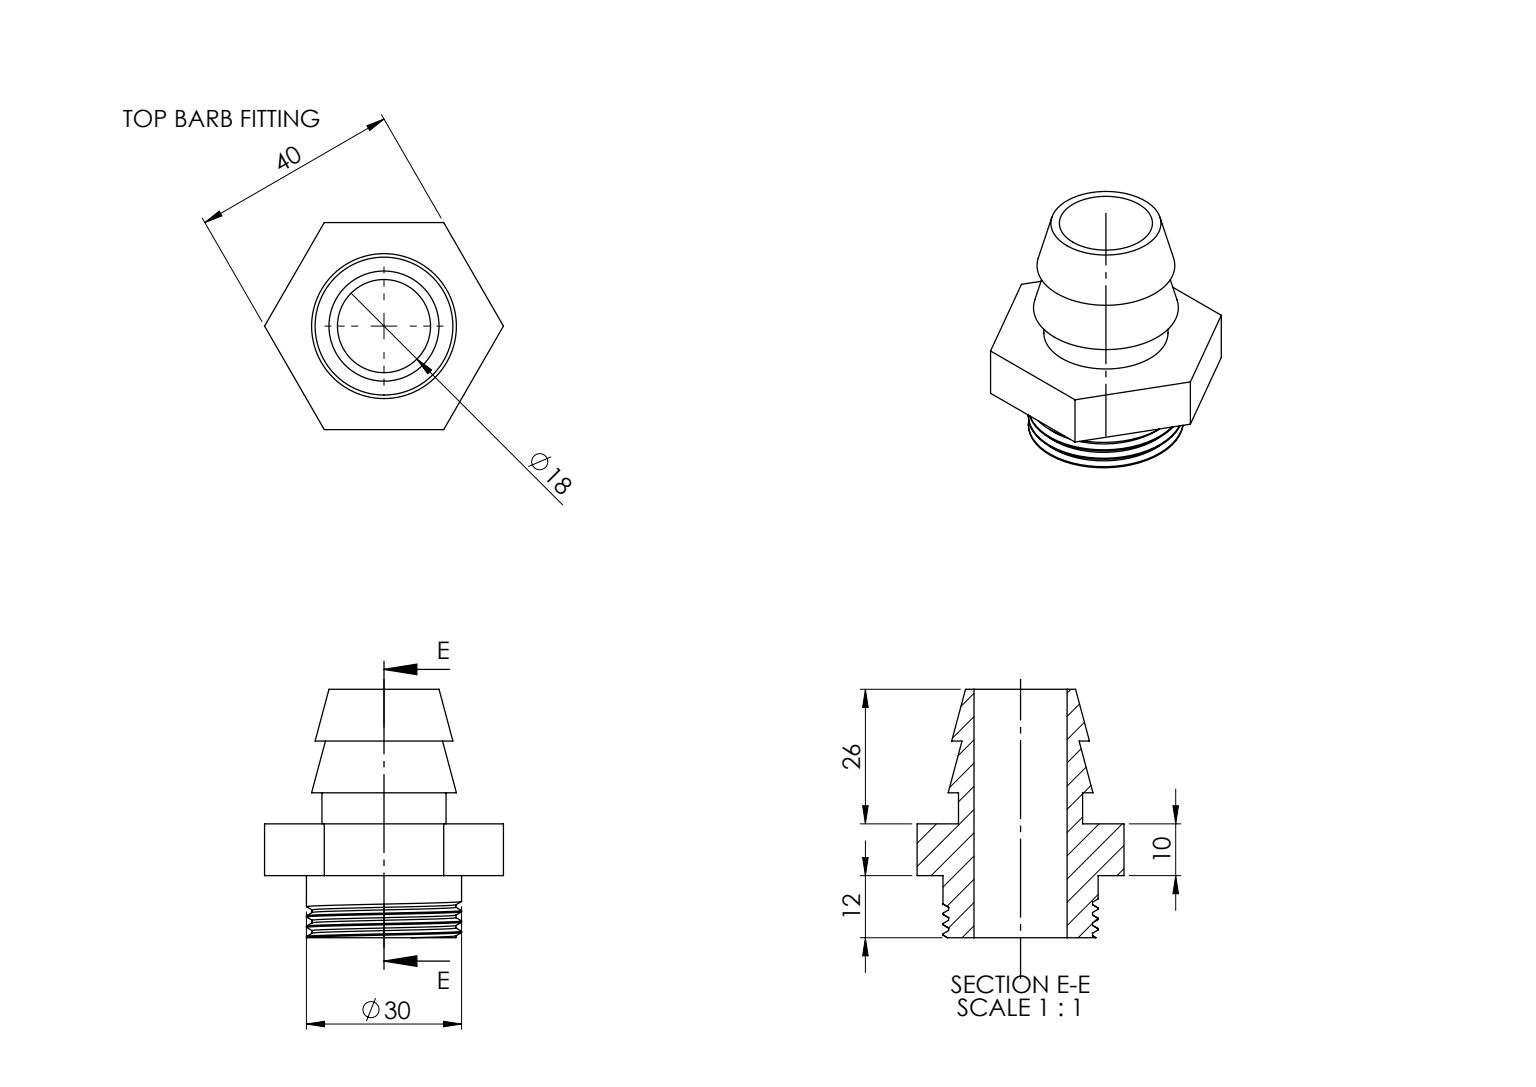
ISO-10303-21;
HEADER;
FILE_DESCRIPTION (('STEP AP214'),
    '1' );
FILE_NAME ('top barb fitting.step',
    '2026-10-02T18:08:48',
    ( '' ),
    ( '' ),
    'SwSTEP 2.0',
    'SolidWorks 2026',
    '' );
FILE_SCHEMA (( 'AUTOMOTIVE_DESIGN' ));
ENDSEC;

DATA;
#6=B_SPLINE_CURVE_WITH_KNOTS ( 'NONE', 3,
 ( #2746, #31563, #23520, #5150, #31895, #33979, #26595, #13563, #7891, #10812, #8061, #21292, #8391, #3092, #18876, #13210, #18378, #13388, #5322, #18546, #24026, #325, #29325, #15802, #5827, #26258, #31732, #495, #23687, #16306, #152, #15636, #2584, #10642 ),
 .UNSPECIFIED., .F., .F.,
 ( 4, 2, 2, 2, 2, 2, 2, 2, 2, 2, 2, 2, 2, 2, 2, 2, 4 ),
 ( 6.762863467562367515E-16, 0.001783076374787156146, 0.003566152749573635750, 0.007132305499146594091, 0.008023843686539834652, 0.008915381873933073478, 0.01069845824871955460, 0.01248153462350603572, 0.01426461099829251858, 0.01604768737307899970, 0.01783076374786548429, 0.02139691649743844307, 0.02228845468483168710, 0.02317999287222492766, 0.02496306924701141225, 0.02674614562179789337, 0.02852922199658437796 ),
 .UNSPECIFIED. ) ;
#9=CARTESIAN_POINT ( 'NONE',  ( -23.09401076758502924, 96.00000000000002842, 5.354274672883389237E-15 ) ) ;
#12=PRODUCT ( 'top barb fitting', 'top barb fitting', '', ( #25356 ) ) ;
#18=CARTESIAN_POINT ( 'NONE',  ( 13.91687918246660871, 74.00000000000008527, 0.9182373085827880699 ) ) ;
#119=DIRECTION ( 'NONE',  ( -0.000000000000000000, 1.000000000000000000, -0.000000000000000000 ) ) ;
#130=EDGE_LOOP ( 'NONE', ( #13807, #32440, #5639, #27881 ) ) ;
#142=CARTESIAN_POINT ( 'NONE',  ( -15.00000000000000000, 72.09999999999999432, 4.873795443493597723 ) ) ;
#152=CARTESIAN_POINT ( 'NONE',  ( 11.86847005202517380, 74.00000000000004263, -7.471229617278120294 ) ) ;
#163=CARTESIAN_POINT ( 'NONE',  ( 8.601468415847520532, 79.57500000273117280, 11.83890561707634603 ) ) ;
#166=CARTESIAN_POINT ( 'NONE',  ( 8.601468415847516980, 76.67500000273118133, -11.83890561707634781 ) ) ;
#187=AXIS2_PLACEMENT_3D ( 'NONE', #2552, #20584, #13357 ) ;
#196=CARTESIAN_POINT ( 'NONE',  ( -1.714505518806294835E-15, 102.0000000000000284, -14.00000000000000178 ) ) ;
#220=VERTEX_POINT ( 'NONE', #33464 ) ;
#287=CARTESIAN_POINT ( 'NONE',  ( 15.00000000000000355, 71.15000000546237402, 4.873795443493592394 ) ) ;
#293=ADVANCED_FACE ( 'NONE', ( #15638 ), #7725, .F. ) ;
#325=CARTESIAN_POINT ( 'NONE',  ( 6.987025175984479475, 74.00000000000002842, -12.51940829596972016 ) ) ;
#333=DIRECTION ( 'NONE',  ( -0.000000000000000000, -1.000000000000000000, -0.000000000000000000 ) ) ;
#335=CARTESIAN_POINT ( 'NONE',  ( 0.000000000000000000, 74.00000000000001421, 0.000000000000000000 ) ) ;
#338=CARTESIAN_POINT ( 'NONE',  ( -4.300734207923759378, 76.47500000273116427, -13.23629886949340495 ) ) ;
#341=CARTESIAN_POINT ( 'NONE',  ( -13.91746824999999887, 75.37500000273116996, 0.000000000000000000 ) ) ;
#357=CARTESIAN_POINT ( 'NONE',  ( -11.25946833292375793, 77.17500000273119554, -8.180482586598733619 ) ) ;
#432=CARTESIAN_POINT ( 'NONE',  ( 1.836970198721029589E-15, 86.00000000000001421, -15.00000000000000000 ) ) ;
#459=CARTESIAN_POINT ( 'NONE',  ( 2.688165632520823219E-15, 79.37500000273116996, 14.63369212191046387 ) ) ;
#486=CARTESIAN_POINT ( 'NONE',  ( -15.00000000000000000, 72.00000000000001421, 0.000000000000000000 ) ) ;
#495=CARTESIAN_POINT ( 'NONE',  ( 10.52536686629071916, 74.00000000000000000, -9.403734997071314439 ) ) ;
#507=CARTESIAN_POINT ( 'NONE',  ( 4.300734207923761154, 77.47500000273116427, 13.23629886949340495 ) ) ;
#510=CARTESIAN_POINT ( 'NONE',  ( 11.25946833292375793, 72.17500000273119554, 8.180482586598731842 ) ) ;
#523=CARTESIAN_POINT ( 'NONE',  ( 11.25946833292375793, 78.17500000273119554, 8.180482586598731842 ) ) ;
#527=CARTESIAN_POINT ( 'NONE',  ( 13.03261263866114206, 74.00000000000001421, 4.904499419084999090 ) ) ;
#550=CARTESIAN_POINT ( 'NONE',  ( -11.25946833292375793, 80.67500000273119554, -8.180482586598733619 ) ) ;
#612=CARTESIAN_POINT ( 'NONE',  ( -1.089172066684569321E-14, 76.75000000546238255, 15.00000000000000000 ) ) ;
#623=CARTESIAN_POINT ( 'NONE',  ( -8.601468415847518756, 78.57500000273120122, -11.83890561707634781 ) ) ;
#647=CARTESIAN_POINT ( 'NONE',  ( 1.836970198721029589E-15, 74.00000000000001421, -15.00000000000000000 ) ) ;
#651=CARTESIAN_POINT ( 'NONE',  ( -12.13525491562420910, 72.19999999999998863, 8.816778784387098611 ) ) ;
#691=CARTESIAN_POINT ( 'NONE',  ( -11.25946833292375793, 79.57500000273121543, 8.180482586598737171 ) ) ;
#716=CARTESIAN_POINT ( 'NONE',  ( -13.91746824999999887, 78.87500000273118417, 0.000000000000000000 ) ) ;
#728=AXIS2_PLACEMENT_3D ( 'NONE', #8070, #26267, #31742 ) ;
#731=LINE ( 'NONE', #16213, #1228 ) ;
#743=ORIENTED_EDGE ( 'NONE', *, *, #12358, .F. ) ;
#754=AXIS2_PLACEMENT_3D ( 'NONE', #32475, #1069, #27509 ) ;
#759=DIRECTION ( 'NONE',  ( -0.000000000000000000, 1.000000000000000000, -0.000000000000000000 ) ) ;
#777=CARTESIAN_POINT ( 'NONE',  ( 15.00000000000000000, 75.35000000546236265, -4.873795443493596835 ) ) ;
#784=CARTESIAN_POINT ( 'NONE',  ( -8.891200544363830713E-16, 77.75000000546235412, -15.00000000000000000 ) ) ;
#792=CARTESIAN_POINT ( 'NONE',  ( 8.601468415847516980, 80.17500000273113869, -11.83890561707634781 ) ) ;
#797=CARTESIAN_POINT ( 'NONE',  ( -15.00000000000000000, 80.15000000546237402, -4.873795443493594171 ) ) ;
#818=COLOUR_RGB ( '', 0.40784314, 0.44705882, 0.49803922) ;
#852=AXIS2_PLACEMENT_3D ( 'NONE', #3223, #24155, #11436 ) ;
#858=CARTESIAN_POINT ( 'NONE',  ( -8.601468415847518756, 81.07500000273115859, -11.83890561707634781 ) ) ;
#865=DIRECTION ( 'NONE',  ( -0.5000000000000002220, 0.000000000000000000, -0.8660254037844384856 ) ) ;
#866=CARTESIAN_POINT ( 'NONE',  ( -11.25946833292375793, 75.57500000273120122, 8.180482586598737171 ) ) ;
#868=FACE_OUTER_BOUND ( 'NONE', #18191, .T. ) ;
#871=VERTEX_POINT ( 'NONE', #20231 ) ;
#874=CARTESIAN_POINT ( 'NONE',  ( -14.45873412499999944, 81.68750000136559208, 0.000000000000000000 ) ) ;
#883=CARTESIAN_POINT ( 'NONE',  ( -11.25946833292375793, 79.07500000273121543, 8.180482586598737171 ) ) ;
#893=EDGE_LOOP ( 'NONE', ( #32042, #24575 ) ) ;
#921=CARTESIAN_POINT ( 'NONE',  ( 0.000000000000000000, 111.9999999999999858, 0.000000000000000000 ) ) ;
#953=CARTESIAN_POINT ( 'NONE',  ( 11.25946833292375793, 75.67500000273119554, 8.180482586598731842 ) ) ;
#1003=CARTESIAN_POINT ( 'NONE',  ( -4.300734207923755825, 71.77500000273117564, 13.23629886949340673 ) ) ;
#1004=DIRECTION ( 'NONE',  ( -0.000000000000000000, -1.000000000000000000, -0.000000000000000000 ) ) ;
#1016=CARTESIAN_POINT ( 'NONE',  ( -12.13525491562421088, 81.79999999999998295, -8.816778784387096835 ) ) ;
#1027=CARTESIAN_POINT ( 'NONE',  ( -13.91746824999999887, 79.37500000273118417, 0.000000000000000000 ) ) ;
#1043=CARTESIAN_POINT ( 'NONE',  ( 8.601468415847520532, 77.57500000273115859, 11.83890561707634781 ) ) ;
#1069=DIRECTION ( 'NONE',  ( 0.000000000000000000, 1.000000000000000000, 0.000000000000000000 ) ) ;
#1099=CARTESIAN_POINT ( 'NONE',  ( 2.375766604868046361, 74.80125428700921475, 14.99999999999999822 ) ) ;
#1105=CARTESIAN_POINT ( 'NONE',  ( -8.891200544363830713E-16, 77.49999999999998579, -15.00000000000000000 ) ) ;
#1113=CARTESIAN_POINT ( 'NONE',  ( -13.91746824999999532, 76.97500000273119269, 4.522059556121122093 ) ) ;
#1186=CARTESIAN_POINT ( 'NONE',  ( 13.91746825000000065, 72.27500000273116143, 4.522059556121114987 ) ) ;
#1196=CARTESIAN_POINT ( 'NONE',  ( -11.25946833292375793, 77.17500000273119554, -8.180482586598733619 ) ) ;
#1210=CARTESIAN_POINT ( 'NONE',  ( -4.300734207923755825, 79.27500000273118985, 13.23629886949340673 ) ) ;
#1228=VECTOR ( 'NONE', #21690, 1000.000000000000114 ) ;
#1250=CARTESIAN_POINT ( 'NONE',  ( -13.91746824999999532, 80.77500000273118985, -4.522059556121115875 ) ) ;
#1253=FILL_AREA_STYLE ('',( #27360 ) ) ;
#1256=ADVANCED_FACE ( 'NONE', ( #33351, #25805 ), #9849, .F. ) ;
#1262=ADVANCED_FACE ( 'NONE', ( #28543, #2297 ), #10028, .T. ) ;
#1269=CARTESIAN_POINT ( 'NONE',  ( -4.635254915624211769, 75.59999999999999432, -14.26584774442730286 ) ) ;
#1285=CARTESIAN_POINT ( 'NONE',  ( -8.601468415847518756, 74.57500000273120122, -11.83890561707634781 ) ) ;
#1300=CLOSED_SHELL ( 'NONE', ( #7560, #13574, #15897, #13035, #6079, #19634, #15027, #28982, #8831, #17642, #33557, #1262, #15751, #14298, #30209, #23775, #26972, #23633, #2088, #3006, #29689, #33907, #4803, #9146, #33895, #7895, #1256, #14876, #293, #28324, #14823, #26573 ) ) ;
#1315=CARTESIAN_POINT ( 'NONE',  ( -3.922490400387641962, 74.00000000000000000, 13.75156615976576902 ) ) ;
#1320=( NAMED_UNIT ( * ) SI_UNIT ( $, .STERADIAN. ) SOLID_ANGLE_UNIT ( ) );
#1338=CARTESIAN_POINT ( 'NONE',  ( -12.13525491562420910, 78.45000000546237118, 8.816778784387098611 ) ) ;
#1348=VECTOR ( 'NONE', #1004, 1000.000000000000000 ) ;
#1358=CARTESIAN_POINT ( 'NONE',  ( -8.960552108402742093E-16, 74.87500000273119838, -14.63369212191046387 ) ) ;
#1368=AXIS2_PLACEMENT_3D ( 'NONE', #32981, #17395, #27514 ) ;
#1370=CARTESIAN_POINT ( 'NONE',  ( -4.300734207923759378, 80.97500000273122112, -13.23629886949340495 ) ) ;
#1372=CARTESIAN_POINT ( 'NONE',  ( -4.635254915624211769, 77.85000000546237686, -14.26584774442730286 ) ) ;
#1376=AXIS2_PLACEMENT_3D ( 'NONE', #6186, #27460, #21818 ) ;
#1387=CARTESIAN_POINT ( 'NONE',  ( 8.601468415847520532, 71.57500000273118701, 11.83890561707634781 ) ) ;
#1437=AXIS2_PLACEMENT_3D ( 'NONE', #30037, #32278, #3798 ) ;
#1459=CARTESIAN_POINT ( 'NONE',  ( 13.91746824999999532, 73.97500000273115006, -4.522059556121118540 ) ) ;
#1470=VECTOR ( 'NONE', #27620, 1000.000000000000000 ) ;
#1509=CARTESIAN_POINT ( 'NONE',  ( -15.00000000000000000, 78.25000000546239676, 0.000000000000000000 ) ) ;
#1517=ORIENTED_EDGE ( 'NONE', *, *, #21552, .F. ) ;
#1530=CARTESIAN_POINT ( 'NONE',  ( 13.91746824999999532, 72.47500000273116427, -4.522059556121118540 ) ) ;
#1541=CARTESIAN_POINT ( 'NONE',  ( 4.635254915624209993, 77.65000000546234560, -14.26584774442730463 ) ) ;
#1553=CARTESIAN_POINT ( 'NONE',  ( -8.960552108402742093E-16, 80.87500000273116996, -14.63369212191046387 ) ) ;
#1624=CARTESIAN_POINT ( 'NONE',  ( 8.601468415847516980, 76.17500000273115290, -11.83890561707634781 ) ) ;
#1644=EDGE_CURVE ( 'NONE', #17496, #30053, #15696, .T. ) ;
#1699=CARTESIAN_POINT ( 'NONE',  ( 4.300734207923757602, 72.77500000273118985, -13.23629886949340673 ) ) ;
#1710=CARTESIAN_POINT ( 'NONE',  ( 12.13525491562421088, 77.05000000546242234, 8.816778784387095058 ) ) ;
#1722=CARTESIAN_POINT ( 'NONE',  ( 4.300734207923757602, 80.77500000273118985, -13.23629886949340673 ) ) ;
#1724=LINE ( 'NONE', #12204, #13775 ) ;
#1792=FACE_OUTER_BOUND ( 'NONE', #13191, .T. ) ;
#1798=CARTESIAN_POINT ( 'NONE',  ( -8.601468415847515203, 71.17500000273118133, 11.83890561707634959 ) ) ;
#1822=CARTESIAN_POINT ( 'NONE',  ( 0.000000000000000000, 102.0000000000000284, 0.000000000000000000 ) ) ;
#1824=VECTOR ( 'NONE', #15914, 1000.000000000000000 ) ;
#1830=CARTESIAN_POINT ( 'NONE',  ( -6.159586018150516651, 74.00000000000001421, 12.99395819748794700 ) ) ;
#1852=CARTESIAN_POINT ( 'NONE',  ( -4.635254915624208216, 78.65000000546234560, 14.26584774442730463 ) ) ;
#1873=CARTESIAN_POINT ( 'NONE',  ( 2.897257156509938333E-15, 74.49999999999995737, 15.77193336357400710 ) ) ;
#1885=CARTESIAN_POINT ( 'NONE',  ( 15.00000000000000000, 75.35000000546236265, -4.873795443493596835 ) ) ;
#1892=CARTESIAN_POINT ( 'NONE',  ( 2.445080149700053643E-15, 74.75000000546239676, 15.00000000000000000 ) ) ;
#1898=CARTESIAN_POINT ( 'NONE',  ( 4.300734207923757602, 80.27500000273118985, -13.23629886949340673 ) ) ;
#1901=CARTESIAN_POINT ( 'NONE',  ( -13.91746824999999532, 74.77500000273118985, -4.522059556121115875 ) ) ;
#1942=EDGE_CURVE ( 'NONE', #22733, #28806, #27713, .T. ) ;
#1950=EDGE_LOOP ( 'NONE', ( #6804, #16249, #16847, #32834 ) ) ;
#1962=CARTESIAN_POINT ( 'NONE',  ( -12.13525491562420910, 76.19999999999998863, 8.816778784387098611 ) ) ;
#1973=DIRECTION ( 'NONE',  ( 0.000000000000000000, 0.000000000000000000, 1.000000000000000000 ) ) ;
#2000=DIRECTION ( 'NONE',  ( -0.000000000000000000, -1.000000000000000000, -0.000000000000000000 ) ) ;
#2041=DIRECTION ( 'NONE',  ( 0.000000000000000000, 0.000000000000000000, 1.000000000000000000 ) ) ;
#2050=CARTESIAN_POINT ( 'NONE',  ( -15.00000000000000000, 76.09999999999999432, 4.873795443493597723 ) ) ;
#2061=CARTESIAN_POINT ( 'NONE',  ( 2.897257156509938333E-15, 74.75000000546236834, 15.77193336357400710 ) ) ;
#2074=CARTESIAN_POINT ( 'NONE',  ( -8.601468415847518756, 72.57500000273114438, -11.83890561707634781 ) ) ;
#2076=B_SPLINE_CURVE_WITH_KNOTS ( 'NONE', 3,
 ( #25351, #32719, #33410, #22780, #11964, #24837, #22603, #15062, #7154, #4074, #33057, #1315, #9562, #22435, #20040, #1830, #12131, #28098, #25178, #14378, #22276, #12308, #20217, #17129, #33232, #30835, #6814, #30485, #30657, #19863, #17637, #11798, #17469, #7327, #32882, #9215 ),
 .UNSPECIFIED., .F., .F.,
 ( 4, 2, 2, 2, 2, 2, 2, 2, 2, 2, 2, 2, 2, 2, 2, 2, 2, 4 ),
 ( 8.685284222369515922E-16, 0.001784781750657605560, 0.003569563501314342892, 0.007139127002627816687, 0.008031517877956187088, 0.008923908753284555753, 0.01070869050394129135, 0.01160108137926966002, 0.01249347225459802868, 0.01427825400525476254, 0.01606303575591149987, 0.01784781750656823027, 0.02141738100788169799, 0.02230977188321005972, 0.02320216275853842838, 0.02498694450919515878, 0.02677172625985189611, 0.02855650801050862303 ),
 .UNSPECIFIED. ) ;
#2088=ADVANCED_FACE ( 'NONE', ( #12555 ), #4312, .F. ) ;
#2203=ORIENTED_EDGE ( 'NONE', *, *, #31596, .T. ) ;
#2215=CARTESIAN_POINT ( 'NONE',  ( -12.13525491562420910, 78.19999999999998863, 8.816778784387098611 ) ) ;
#2221=EDGE_CURVE ( 'NONE', #6130, #17496, #29511, .T. ) ;
#2227=CARTESIAN_POINT ( 'NONE',  ( -8.960552108402744065E-16, 74.87500000273119838, -14.63369212191046209 ) ) ;
#2229=CARTESIAN_POINT ( 'NONE',  ( 4.300734207923757602, 80.27500000273118985, -13.23629886949340673 ) ) ;
#2230=EDGE_CURVE ( 'NONE', #17496, #8542, #20976, .T. ) ;
#2236=CARTESIAN_POINT ( 'NONE',  ( -11.43271046912435196, 74.02547620226849290, -9.783748258876929782 ) ) ;
#2245=CARTESIAN_POINT ( 'NONE',  ( 8.601468415847516980, 74.67500000273120975, -11.83890561707634781 ) ) ;
#2297=FACE_OUTER_BOUND ( 'NONE', #130, .T. ) ;
#2316=CARTESIAN_POINT ( 'NONE',  ( 9.270509831248425314, 80.69999999999998863, 12.75976212528059683 ) ) ;
#2352=DIRECTION ( 'NONE',  ( 0.000000000000000000, -0.000000000000000000, 1.000000000000000000 ) ) ;
#2390=ORIENTED_EDGE ( 'NONE', *, *, #16303, .F. ) ;
#2397=CARTESIAN_POINT ( 'NONE',  ( 9.270509831248425314, 76.70000000000003126, 12.75976212528059683 ) ) ;
#2409=CARTESIAN_POINT ( 'NONE',  ( 4.300734207923757602, 74.77500000273118985, -13.23629886949340673 ) ) ;
#2419=CARTESIAN_POINT ( 'NONE',  ( -8.601468415847515203, 79.17500000273116711, 11.83890561707634959 ) ) ;
#2422=CARTESIAN_POINT ( 'NONE',  ( -11.25946833292375793, 75.57500000273120122, 8.180482586598737171 ) ) ;
#2440=CARTESIAN_POINT ( 'NONE',  ( -4.635254915624208216, 76.65000000546234560, 14.26584774442730463 ) ) ;
#2515=CIRCLE ( 'NONE', #852, 12.00000000000000000 ) ;
#2552=CARTESIAN_POINT ( 'NONE',  ( 0.000000000000000000, 102.0000000000000284, 0.000000000000000000 ) ) ;
#2573=CARTESIAN_POINT ( 'NONE',  ( 15.00000000000000355, 74.90000000000003411, 4.873795443493592394 ) ) ;
#2578=AXIS2_PLACEMENT_3D ( 'NONE', #30953, #25809, #17935 ) ;
#2584=CARTESIAN_POINT ( 'NONE',  ( 12.65897589331677153, 74.00000000000004263, -5.871086419100934428 ) ) ;
#2594=CARTESIAN_POINT ( 'NONE',  ( 4.300734207923761154, 79.47500000273116427, 13.23629886949340495 ) ) ;
#2597=CARTESIAN_POINT ( 'NONE',  ( -13.91746824999999532, 77.27500000273117564, -4.522059556121115875 ) ) ;
#2626=CARTESIAN_POINT ( 'NONE',  ( -11.54700538379251817, 96.00000000000002842, 19.99999999999999645 ) ) ;
#2665=CARTESIAN_POINT ( 'NONE',  ( 9.270509831248421762, 81.29999999999999716, -12.75976212528059861 ) ) ;
#2701=DIRECTION ( 'NONE',  ( 0.000000000000000000, 1.000000000000000000, 0.000000000000000000 ) ) ;
#2746=CARTESIAN_POINT ( 'NONE',  ( -10.58590195883389207, 74.00000000000001421, -10.62726115788808201 ) ) ;
#2756=CARTESIAN_POINT ( 'NONE',  ( 2.688165632520823219E-15, 75.37500000273118417, 14.63369212191046209 ) ) ;
#2760=CARTESIAN_POINT ( 'NONE',  ( 11.25946833292375793, 76.57500000273120122, -8.180482586598735395 ) ) ;
#2774=DIRECTION ( 'NONE',  ( -0.000000000000000000, -1.000000000000000000, -0.000000000000000000 ) ) ;
#2777=CARTESIAN_POINT ( 'NONE',  ( -13.91746824999999532, 77.47500000273117848, 4.522059556121122093 ) ) ;
#2808=ORIENTED_EDGE ( 'NONE', *, *, #26669, .F. ) ;
#2820=DIRECTION ( 'NONE',  ( 0.000000000000000000, -1.000000000000000000, 0.000000000000000000 ) ) ;
#2822=EDGE_CURVE ( 'NONE', #4956, #8605, #4255, .T. ) ;
#2881=AXIS2_PLACEMENT_3D ( 'NONE', #29621, #3394, #6124 ) ;
#2882=CARTESIAN_POINT ( 'NONE',  ( -9.270509831248425314, 71.95000000546239960, -12.75976212528059861 ) ) ;
#2929=VECTOR ( 'NONE', #28226, 1000.000000000000000 ) ;
#2930=CARTESIAN_POINT ( 'NONE',  ( 8.601468415847516980, 78.17500000273120975, -11.83890561707634603 ) ) ;
#2933=CARTESIAN_POINT ( 'NONE',  ( -4.300734207923755825, 75.77500000273118985, 13.23629886949340673 ) ) ;
#2947=CARTESIAN_POINT ( 'NONE',  ( -13.91746824999999532, 77.27500000273117564, -4.522059556121115875 ) ) ;
#2985=CARTESIAN_POINT ( 'NONE',  ( 15.00000000000000355, 76.90000000000000568, 4.873795443493592394 ) ) ;
#3006=ADVANCED_FACE ( 'NONE', ( #8379 ), #3078, .F. ) ;
#3053=CARTESIAN_POINT ( 'NONE',  ( -8.601468415847515203, 79.17500000273116711, 11.83890561707634959 ) ) ;
#3078=PLANE ( 'NONE',  #11914 ) ;
#3092=CARTESIAN_POINT ( 'NONE',  ( -0.3491184494335538013, 73.99999999999998579, -14.58811049051102415 ) ) ;
#3104=CARTESIAN_POINT ( 'NONE',  ( 4.300734207923757602, 78.27500000273118985, -13.23629886949340673 ) ) ;
#3107=CARTESIAN_POINT ( 'NONE',  ( -11.25946833292375793, 73.17500000273119554, -8.180482586598733619 ) ) ;
#3120=CARTESIAN_POINT ( 'NONE',  ( 2.688165632520823219E-15, 75.87500000273115575, 14.63369212191046387 ) ) ;
#3123=CARTESIAN_POINT ( 'NONE',  ( 0.000000000000000000, 111.9999999999999858, 0.000000000000000000 ) ) ;
#3134=ORIENTED_EDGE ( 'NONE', *, *, #25934, .T. ) ;
#3157=EDGE_CURVE ( 'NONE', #9414, #21926, #16291, .T. ) ;
#3201=FACE_OUTER_BOUND ( 'NONE', #9127, .T. ) ;
#3220=CARTESIAN_POINT ( 'NONE',  ( -9.270509831248421762, 72.55000000546239391, 12.75976212528060039 ) ) ;
#3223=CARTESIAN_POINT ( 'NONE',  ( 0.000000000000000000, 96.00000000000002842, 0.000000000000000000 ) ) ;
#3225=DIRECTION ( 'NONE',  ( 0.000000000000000000, 1.000000000000000000, 0.000000000000000000 ) ) ;
#3237=ORIENTED_EDGE ( 'NONE', *, *, #17210, .F. ) ;
#3245=CARTESIAN_POINT ( 'NONE',  ( -9.270509831248421762, 72.29999999999999716, 12.75976212528060039 ) ) ;
#3263=CARTESIAN_POINT ( 'NONE',  ( 11.54700538379251107, 96.00000000000002842, -19.99999999999999645 ) ) ;
#3268=SHAPE_REPRESENTATION ( 'top barb fitting', ( #1376 ), #19430 ) ;
#3277=EDGE_CURVE ( 'NONE', #5214, #19151, #20139, .T. ) ;
#3282=CARTESIAN_POINT ( 'NONE',  ( 8.601468415847520532, 80.07500000273120122, 11.83890561707634781 ) ) ;
#3286=CARTESIAN_POINT ( 'NONE',  ( 11.07021743829117710, 74.00000000000002842, 8.483650685288816717 ) ) ;
#3311=CARTESIAN_POINT ( 'NONE',  ( 13.91746824999999887, 75.87500000273116996, -1.704398294459741270E-15 ) ) ;
#3373=CARTESIAN_POINT ( 'NONE',  ( 15.00000000000000000, 77.25000000546239676, -1.836970198721029589E-15 ) ) ;
#3383=CARTESIAN_POINT ( 'NONE',  ( -4.300734207923759378, 78.47500000273116427, -13.23629886949340495 ) ) ;
#3394=DIRECTION ( 'NONE',  ( -0.000000000000000000, 1.000000000000000000, -0.000000000000000000 ) ) ;
#3437=AXIS2_PLACEMENT_3D ( 'NONE', #6769, #30611, #7107 ) ;
#3473=CARTESIAN_POINT ( 'NONE',  ( -13.91746824999999887, 76.87500000273116996, 0.000000000000000000 ) ) ;
#3544=CARTESIAN_POINT ( 'NONE',  ( -4.300734207923759378, 76.47500000273116427, -13.23629886949340495 ) ) ;
#3550=CARTESIAN_POINT ( 'NONE',  ( -15.00000000000000000, 80.10000000000003695, 4.873795443493597723 ) ) ;
#3598=CARTESIAN_POINT ( 'NONE',  ( -13.91746824999999887, 71.37500000273116996, 0.000000000000000000 ) ) ;
#3614=CARTESIAN_POINT ( 'NONE',  ( 15.00000000000000000, 81.00000000000001421, -1.836970198721029589E-15 ) ) ;
#3624=CARTESIAN_POINT ( 'NONE',  ( -11.25946833292375793, 81.17500000273119554, -8.180482586598733619 ) ) ;
#3665=CIRCLE ( 'NONE', #23090, 14.00000000000000178 ) ;
#3690=VECTOR ( 'NONE', #31924, 1000.000000000000000 ) ;
#3692=DIRECTION ( 'NONE',  ( 0.000000000000000000, -0.000000000000000000, 1.000000000000000000 ) ) ;
#3696=CARTESIAN_POINT ( 'NONE',  ( 2.375766604868043252, 75.69874572391552192, -14.99999999999999822 ) ) ;
#3713=CARTESIAN_POINT ( 'NONE',  ( -8.960552108402742093E-16, 76.37500000273114154, -14.63369212191046387 ) ) ;
#3743=DIRECTION ( 'NONE',  ( 0.000000000000000000, 1.000000000000000000, 0.000000000000000000 ) ) ;
#3774=VERTEX_POINT ( 'NONE', #11060 ) ;
#3781=CARTESIAN_POINT ( 'NONE',  ( 4.300734207923757602, 74.77500000273118985, -13.23629886949340673 ) ) ;
#3791=CARTESIAN_POINT ( 'NONE',  ( -8.601468415847515203, 79.67500000273115290, 11.83890561707634959 ) ) ;
#3794=ORIENTED_EDGE ( 'NONE', *, *, #7358, .F. ) ;
#3798=DIRECTION ( 'NONE',  ( 0.000000000000000000, 0.000000000000000000, 1.000000000000000000 ) ) ;
#3807=CARTESIAN_POINT ( 'NONE',  ( -4.300734207923755825, 77.27500000273118985, 13.23629886949340673 ) ) ;
#3832=ORIENTED_EDGE ( 'NONE', *, *, #7432, .T. ) ;
#3877=CARTESIAN_POINT ( 'NONE',  ( -13.91746824999999532, 76.77500000273118985, -4.522059556121115875 ) ) ;
#3947=CARTESIAN_POINT ( 'NONE',  ( 9.270509831248425314, 80.70000000000000284, 12.75976212528059683 ) ) ;
#3957=CARTESIAN_POINT ( 'NONE',  ( 4.300734207923757602, 80.77500000273118985, -13.23629886949340673 ) ) ;
#3959=CARTESIAN_POINT ( 'NONE',  ( -9.270509831248425314, 79.95000000546238539, -12.75976212528059861 ) ) ;
#3973=CARTESIAN_POINT ( 'NONE',  ( -11.25946833292375793, 72.67500000273119554, -8.180482586598733619 ) ) ;
#4043=CARTESIAN_POINT ( 'NONE',  ( 4.300734207923757602, 78.27500000273118985, -13.23629886949340673 ) ) ;
#4064=VERTEX_POINT ( 'NONE', #31183 ) ;
#4074=CARTESIAN_POINT ( 'NONE',  ( -2.762933978968158399, 73.99999999999998579, 13.97530310184241031 ) ) ;
#4095=CARTESIAN_POINT ( 'NONE',  ( -15.00000000000000000, 78.15000000546238823, -4.873795443493594171 ) ) ;
#4116=CARTESIAN_POINT ( 'NONE',  ( 12.13525491562421088, 80.79999999999998295, 8.816778784387095058 ) ) ;
#4128=CARTESIAN_POINT ( 'NONE',  ( -15.00000000000000000, 74.25000000546239676, 0.000000000000000000 ) ) ;
#4133=CARTESIAN_POINT ( 'NONE',  ( -10.58590195883389207, 74.00000000000001421, -10.62726115788808201 ) ) ;
#4141=CARTESIAN_POINT ( 'NONE',  ( -4.300734207923755825, 71.27500000273117564, 13.23629886949340673 ) ) ;
#4172=VERTEX_POINT ( 'NONE', #17814 ) ;
#4215=CARTESIAN_POINT ( 'NONE',  ( -11.25946833292375793, 72.67500000273119554, -8.180482586598733619 ) ) ;
#4231=VERTEX_POINT ( 'NONE', #21200 ) ;
#4255=( BOUNDED_CURVE ( )  B_SPLINE_CURVE ( 2, ( #25567, #31216, #7709, #30525, #23160, #7023, #33623, #9771, #22990, #25393, #33449, #10122, #12348 ),
 .UNSPECIFIED., .F., .T. ) 
 B_SPLINE_CURVE_WITH_KNOTS ( ( 3, 2, 2, 2, 2, 2, 3 ),
 ( 0.05000000000000000278, 0.05999999999999999778, 0.08000000000000000167, 0.1000000000000000056, 0.1199999999999999956, 0.1400000000000000133, 0.1500000000000000222 ),
 .UNSPECIFIED. ) 
 CURVE ( )  GEOMETRIC_REPRESENTATION_ITEM ( )  RATIONAL_B_SPLINE_CURVE ( ( 0.9755282581475768211, 0.9755282581475768211, 1.000000000000000000, 0.9510565162951535312, 1.000000000000000000, 0.9510565162951535312, 1.000000000000000000, 0.9510565162951535312, 1.000000000000000000, 0.9510565162951535312, 1.000000000000000000, 0.9755282581475767101, 0.9755282581475768211 ) ) 
 REPRESENTATION_ITEM ( '' )  );
#4284=CARTESIAN_POINT ( 'NONE',  ( 4.300734207923761154, 73.97500000273122112, 13.23629886949340495 ) ) ;
#4293=CARTESIAN_POINT ( 'NONE',  ( -4.300734207923755825, 75.77500000273118985, 13.23629886949340673 ) ) ;
#4295=CARTESIAN_POINT ( 'NONE',  ( -9.270509831248425314, 75.95000000546238539, -12.75976212528059861 ) ) ;
#4307=CARTESIAN_POINT ( 'NONE',  ( 13.91746824999999532, 80.47500000273119269, -4.522059556121118540 ) ) ;
#4312=PLANE ( 'NONE',  #30523 ) ;
#4364=CARTESIAN_POINT ( 'NONE',  ( 2.445080149700053643E-15, 74.49999999999998579, 15.00000000000000000 ) ) ;
#4402=ORIENTED_EDGE ( 'NONE', *, *, #17994, .F. ) ;
#4440=VERTEX_POINT ( 'NONE', #14732 ) ;
#4453=CARTESIAN_POINT ( 'NONE',  ( -12.13525491562420910, 76.19999999999998863, 8.816778784387098611 ) ) ;
#4466=CARTESIAN_POINT ( 'NONE',  ( -13.91746824999999887, 75.37500000273116996, 0.000000000000000000 ) ) ;
#4468=CARTESIAN_POINT ( 'NONE',  ( -15.00000000000000000, 76.35000000546239107, 4.873795443493597723 ) ) ;
#4481=CARTESIAN_POINT ( 'NONE',  ( -13.91746824999999532, 72.97500000273120691, 4.522059556121122093 ) ) ;
#4565=CARTESIAN_POINT ( 'NONE',  ( -12.13525491562421088, 77.80000000000003979, -8.816778784387096835 ) ) ;
#4614=ORIENTED_EDGE ( 'NONE', *, *, #1942, .F. ) ;
#4626=CARTESIAN_POINT ( 'NONE',  ( 12.13525491562420910, 77.19999999999998863, -8.816778784387098611 ) ) ;
#4636=CARTESIAN_POINT ( 'NONE',  ( 13.91746825000000065, 74.27500000273121827, 4.522059556121115875 ) ) ;
#4638=CARTESIAN_POINT ( 'NONE',  ( 12.13525491562420910, 75.45000000546237118, -8.816778784387098611 ) ) ;
#4652=CARTESIAN_POINT ( 'NONE',  ( -8.601468415847515203, 71.17500000273118133, 11.83890561707634959 ) ) ;
#4657=DIRECTION ( 'NONE',  ( 0.8660254037844387076, 0.000000000000000000, -0.5000000000000001110 ) ) ;
#4707=VECTOR ( 'NONE', #8638, 1000.000000000000000 ) ;
#4732=CARTESIAN_POINT ( 'NONE',  ( -9.270509831248419985, 78.29999999999995453, 12.75976212528060039 ) ) ;
#4738=EDGE_CURVE ( 'NONE', #15262, #16782, #4771, .T. ) ;
#4760=CIRCLE ( 'NONE', #1437, 12.00000000000000178 ) ;
#4771=LINE ( 'NONE', #18173, #31665 ) ;
#4775=DIRECTION ( 'NONE',  ( 0.000000000000000000, 1.000000000000000000, 0.000000000000000000 ) ) ;
#4796=CARTESIAN_POINT ( 'NONE',  ( -15.00000000000000000, 76.00000000000001421, 0.000000000000000000 ) ) ;
#4803=ADVANCED_FACE ( 'NONE', ( #13014 ), #8661, .T. ) ;
#4806=CARTESIAN_POINT ( 'NONE',  ( -13.91746824999999532, 75.27500000273118985, -4.522059556121115875 ) ) ;
#4808=CARTESIAN_POINT ( 'NONE',  ( 15.00000000000000000, 71.35000000546237686, -4.873795443493596835 ) ) ;
#4821=CARTESIAN_POINT ( 'NONE',  ( -4.300734207923759378, 78.97500000273122112, -13.23629886949340495 ) ) ;
#4947=EDGE_CURVE ( 'NONE', #3774, #4956, #20518, .T. ) ;
#4956=VERTEX_POINT ( 'NONE', #18846 ) ;
#4965=EDGE_CURVE ( 'NONE', #29760, #12253, #15816, .T. ) ;
#4971=CARTESIAN_POINT ( 'NONE',  ( -9.270509831248425314, 79.69999999999997442, -12.75976212528059861 ) ) ;
#4990=CARTESIAN_POINT ( 'NONE',  ( -4.300734207923759378, 74.47500000273116427, -13.23629886949340495 ) ) ;
#4993=CARTESIAN_POINT ( 'NONE',  ( 2.688165632520823219E-15, 75.87500000273115575, 14.63369212191046387 ) ) ;
#5010=AXIS2_PLACEMENT_3D ( 'NONE', #25727, #31041, #28299 ) ;
#5060=CARTESIAN_POINT ( 'NONE',  ( 4.635254915624212657, 80.60000000000000853, 14.26584774442730286 ) ) ;
#5097=AXIS2_PLACEMENT_3D ( 'NONE', #18673, #13518, #29283 ) ;
#5104=VECTOR ( 'NONE', #7934, 1000.000000000000000 ) ;
#5138=CARTESIAN_POINT ( 'NONE',  ( -9.270509831248421762, 74.29999999999999716, 12.75976212528060039 ) ) ;
#5150=CARTESIAN_POINT ( 'NONE',  ( -8.724778166670336788, 73.99999999999997158, -12.10690039861944278 ) ) ;
#5161=CARTESIAN_POINT ( 'NONE',  ( -11.25946833292375793, 76.67500000273119554, -8.180482586598733619 ) ) ;
#5164=CARTESIAN_POINT ( 'NONE',  ( -13.91746824999999532, 77.47500000273117848, 4.522059556121122093 ) ) ;
#5214=VERTEX_POINT ( 'NONE', #19179 ) ;
#5233=DIRECTION ( 'NONE',  ( 0.000000000000000000, 0.000000000000000000, 1.000000000000000000 ) ) ;
#5300=EDGE_LOOP ( 'NONE', ( #25430, #32275, #16038, #33271 ) ) ;
#5306=DIRECTION ( 'NONE',  ( -0.000000000000000000, 1.000000000000000000, -0.000000000000000000 ) ) ;
#5322=CARTESIAN_POINT ( 'NONE',  ( 3.730319287574177523, 74.00000000000004263, -13.94370120449079842 ) ) ;
#5331=PLANE ( 'NONE',  #15000 ) ;
#5332=CARTESIAN_POINT ( 'NONE',  ( 13.91746825000000065, 75.77500000273117564, 4.522059556121115875 ) ) ;
#5335=CARTESIAN_POINT ( 'NONE',  ( -11.25946833292375793, 77.57500000273121543, 8.180482586598737171 ) ) ;
#5355=CYLINDRICAL_SURFACE ( 'NONE', #32079, 9.000000000000001776 ) ;
#5433=LINE ( 'NONE', #13672, #1824 ) ;
#5452=CARTESIAN_POINT ( 'NONE',  ( -9.270509831248421762, 70.55000000546240813, 12.75976212528060039 ) ) ;
#5472=EDGE_LOOP ( 'NONE', ( #1517, #25728 ) ) ;
#5502=CARTESIAN_POINT ( 'NONE',  ( 11.25946833292375793, 80.07500000273121543, -8.180482586598735395 ) ) ;
#5505=CARTESIAN_POINT ( 'NONE',  ( -4.300734207923759378, 76.97500000273122112, -13.23629886949340495 ) ) ;
#5521=CARTESIAN_POINT ( 'NONE',  ( -4.300734207923755825, 79.77500000273118985, 13.23629886949340673 ) ) ;
#5562=ORIENTED_EDGE ( 'NONE', *, *, #20203, .F. ) ;
#5592=VERTEX_POINT ( 'NONE', #26531 ) ;
#5622=CARTESIAN_POINT ( 'NONE',  ( 4.635254915624212657, 72.85000000546237686, 14.26584774442730286 ) ) ;
#5632=DIRECTION ( 'NONE',  ( 0.000000000000000000, 1.000000000000000000, 0.000000000000000000 ) ) ;
#5639=ORIENTED_EDGE ( 'NONE', *, *, #10703, .T. ) ;
#5673=CARTESIAN_POINT ( 'NONE',  ( 4.300734207923757602, 76.27500000273118985, -13.23629886949340673 ) ) ;
#5676=CARTESIAN_POINT ( 'NONE',  ( 4.300734207923757602, 72.77500000273118985, -13.23629886949340673 ) ) ;
#5684=VERTEX_POINT ( 'NONE', #432 ) ;
#5691=CARTESIAN_POINT ( 'NONE',  ( 4.300734207923757602, 80.77500000273118985, -13.23629886949340673 ) ) ;
#5693=CARTESIAN_POINT ( 'NONE',  ( -2.375766604868048137, 76.69874572391550771, 14.99999999999999822 ) ) ;
#5726=CARTESIAN_POINT ( 'NONE',  ( 2.375766604868046361, 76.55125428154686062, 14.99999999999999822 ) ) ;
#5779=CARTESIAN_POINT ( 'NONE',  ( 9.270509831248421762, 77.55000000546235128, -12.75976212528059861 ) ) ;
#5787=CARTESIAN_POINT ( 'NONE',  ( -9.270509831248425314, 73.95000000546235697, -12.75976212528059861 ) ) ;
#5819=CARTESIAN_POINT ( 'NONE',  ( -23.09401076758502924, 86.00000000000001421, 5.354274672883389237E-15 ) ) ;
#5827=CARTESIAN_POINT ( 'NONE',  ( 9.299350884854096222, 74.00000000000000000, -10.69806180658744310 ) ) ;
#5842=CARTESIAN_POINT ( 'NONE',  ( -8.960552108402742093E-16, 72.87500000273118417, -14.63369212191046387 ) ) ;
#5856=CARTESIAN_POINT ( 'NONE',  ( 13.91746824999999532, 80.47500000273119269, -4.522059556121118540 ) ) ;
#5883=CARTESIAN_POINT ( 'NONE',  ( 11.25946833292375793, 76.07500000273120122, -8.180482586598735395 ) ) ;
#5929=ORIENTED_EDGE ( 'NONE', *, *, #25577, .T. ) ;
#5938=CARTESIAN_POINT ( 'NONE',  ( 15.00000000000000000, 75.25000000546239676, -1.836970198721029589E-15 ) ) ;
#5954=CARTESIAN_POINT ( 'NONE',  ( 11.25946833292375793, 79.67500000273119554, 8.180482586598731842 ) ) ;
#5961=CARTESIAN_POINT ( 'NONE',  ( 0.000000000000000000, 102.0000000000000284, -9.000000000000001776 ) ) ;
#6004=CARTESIAN_POINT ( 'NONE',  ( 13.91746824999999532, 72.47500000273116427, -4.522059556121118540 ) ) ;
#6010=CARTESIAN_POINT ( 'NONE',  ( 0.000000000000000000, 86.00000000000001421, 15.00000000000000000 ) ) ;
#6018=FACE_OUTER_BOUND ( 'NONE', #20548, .T. ) ;
#6078=DIRECTION ( 'NONE',  ( 0.000000000000000000, 1.000000000000000000, 0.000000000000000000 ) ) ;
#6079=ADVANCED_FACE ( 'NONE', ( #20329 ), #33529, .T. ) ;
#6113=CARTESIAN_POINT ( 'NONE',  ( 13.91746824999999532, 77.97500000273122112, -4.522059556121118540 ) ) ;
#6124=DIRECTION ( 'NONE',  ( 0.000000000000000000, 0.000000000000000000, 1.000000000000000000 ) ) ;
#6130=VERTEX_POINT ( 'NONE', #33876 ) ;
#6168=LINE ( 'NONE', #16819, #1348 ) ;
#6182=CARTESIAN_POINT ( 'NONE',  ( 13.91746824999999887, 78.37500000273116996, -1.704398294459741270E-15 ) ) ;
#6186=CARTESIAN_POINT ( 'NONE',  ( 0.000000000000000000, 0.000000000000000000, 0.000000000000000000 ) ) ;
#6192=CARTESIAN_POINT ( 'NONE',  ( 8.601468415847516980, 78.67500000273119554, -11.83890561707634603 ) ) ;
#6197=ORIENTED_EDGE ( 'NONE', *, *, #27503, .F. ) ;
#6208=CARTESIAN_POINT ( 'NONE',  ( -4.300734207923759378, 78.47500000273116427, -13.23629886949340495 ) ) ;
#6223=ORIENTED_EDGE ( 'NONE', *, *, #19302, .T. ) ;
#6267=( BOUNDED_CURVE ( )  B_SPLINE_CURVE ( 2, ( #22391, #19993, #25483, #12086, #1962, #14671, #24790, #11749, #30441, #32674, #1269, #32840, #17080 ),
 .UNSPECIFIED., .F., .T. ) 
 B_SPLINE_CURVE_WITH_KNOTS ( ( 3, 2, 2, 2, 2, 2, 3 ),
 ( 0.5500000000000000444, 0.5600000000000000533, 0.5799999999999999600, 0.5999999999999999778, 0.6199999999999999956, 0.6400000000000000133, 0.6500000000000000222 ),
 .UNSPECIFIED. ) 
 CURVE ( )  GEOMETRIC_REPRESENTATION_ITEM ( )  RATIONAL_B_SPLINE_CURVE ( ( 0.9755282581475768211, 0.9755282581475768211, 1.000000000000000000, 0.9510565162951535312, 1.000000000000000000, 0.9510565162951535312, 1.000000000000000000, 0.9510565162951535312, 1.000000000000000000, 0.9510565162951535312, 1.000000000000000000, 0.9755282581475768211, 0.9755282581475768211 ) ) 
 REPRESENTATION_ITEM ( '' )  );
#6285=CARTESIAN_POINT ( 'NONE',  ( -13.91746824999999887, 74.87500000273116996, 0.000000000000000000 ) ) ;
#6321=( LENGTH_UNIT ( ) NAMED_UNIT ( * ) SI_UNIT ( .MILLI., .METRE. ) );
#6355=CARTESIAN_POINT ( 'NONE',  ( -8.601468415847518756, 73.07500000273118701, -11.83890561707634781 ) ) ;
#6365=CARTESIAN_POINT ( 'NONE',  ( 13.91746825000000065, 80.27500000273120406, 4.522059556121115875 ) ) ;
#6441=CARTESIAN_POINT ( 'NONE',  ( 15.00000000000000355, 75.15000000546237402, 4.873795443493592394 ) ) ;
#6456=CARTESIAN_POINT ( 'NONE',  ( 2.688165632520823219E-15, 77.37500000273118417, 14.63369212191046387 ) ) ;
#6503=CYLINDRICAL_SURFACE ( 'NONE', #17697, 15.00000000000000000 ) ;
#6526=CARTESIAN_POINT ( 'NONE',  ( -11.25946833292375793, 75.17500000273119554, -8.180482586598733619 ) ) ;
#6536=CARTESIAN_POINT ( 'NONE',  ( 8.601468415847520532, 78.07500000273121543, 11.83890561707634603 ) ) ;
#6550=CARTESIAN_POINT ( 'NONE',  ( 4.300734207923761154, 79.47500000273116427, 13.23629886949340495 ) ) ;
#6564=EDGE_CURVE ( 'NONE', #9414, #22980, #24018, .T. ) ;
#6618=CARTESIAN_POINT ( 'NONE',  ( -13.91746824999999532, 74.77500000273118985, -4.522059556121115875 ) ) ;
#6640=AXIS2_PLACEMENT_3D ( 'NONE', #6647, #8884, #22275 ) ;
#6647=CARTESIAN_POINT ( 'NONE',  ( 0.000000000000000000, 102.0000000000000284, 0.000000000000000000 ) ) ;
#6668=DIRECTION ( 'NONE',  ( 0.000000000000000000, -1.000000000000000000, 0.000000000000000000 ) ) ;
#6687=CARTESIAN_POINT ( 'NONE',  ( -8.960552108402742093E-16, 72.87500000273118417, -14.63369212191046387 ) ) ;
#6697=CARTESIAN_POINT ( 'NONE',  ( -13.91746824999999532, 77.27500000273118985, -4.522059556121115875 ) ) ;
#6699=CARTESIAN_POINT ( 'NONE',  ( 12.13525491562421088, 75.05000000546240813, 8.816778784387095058 ) ) ;
#6714=CARTESIAN_POINT ( 'NONE',  ( -8.960552108402742093E-16, 72.37500000273115575, -14.63369212191046387 ) ) ;
#6769=CARTESIAN_POINT ( 'NONE',  ( 11.54700538379251107, 96.00000000000002842, -19.99999999999999645 ) ) ;
#6778=AXIS2_PLACEMENT_3D ( 'NONE', #20788, #21295, #8063 ) ;
#6786=CARTESIAN_POINT ( 'NONE',  ( 13.91746824999999532, 75.97500000273116427, -4.522059556121118540 ) ) ;
#6804=ORIENTED_EDGE ( 'NONE', *, *, #7993, .F. ) ;
#6814=CARTESIAN_POINT ( 'NONE',  ( -13.36811651448714677, 74.00000000000004263, 6.258549183928298731 ) ) ;
#6858=CARTESIAN_POINT ( 'NONE',  ( -8.601468415847515203, 75.67500000273116711, 11.83890561707634959 ) ) ;
#6867=CARTESIAN_POINT ( 'NONE',  ( 8.601468415847520532, 76.07500000273117280, 11.83890561707634603 ) ) ;
#6880=CARTESIAN_POINT ( 'NONE',  ( -4.300734207923755825, 73.27500000273118985, 13.23629886949340673 ) ) ;
#6906=CARTESIAN_POINT ( 'NONE',  ( -1.631291757790872152E-15, 111.9999999999999858, -13.32050807568876927 ) ) ;
#6937=EDGE_LOOP ( 'NONE', ( #17456, #13462, #25125, #30216 ) ) ;
#6954=CARTESIAN_POINT ( 'NONE',  ( -13.91746824999999887, 70.87500000273122680, 0.000000000000000000 ) ) ;
#7023=CARTESIAN_POINT ( 'NONE',  ( 15.00000000000000000, 79.35000000546240528, -4.873795443493596835 ) ) ;
#7026=CARTESIAN_POINT ( 'NONE',  ( 9.270509831248423538, 81.29999999999999716, -12.75976212528059861 ) ) ;
#7037=CARTESIAN_POINT ( 'NONE',  ( -15.00000000000000000, 80.15000000546237402, -4.873795443493594171 ) ) ;
#7051=CARTESIAN_POINT ( 'NONE',  ( 8.601468415847516980, 74.17500000273122396, -11.83890561707634781 ) ) ;
#7055=CARTESIAN_POINT ( 'NONE',  ( 2.375766604868043252, 79.44874571845312516, -14.99999999999999822 ) ) ;
#7107=DIRECTION ( 'NONE',  ( 1.000000000000000000, 0.000000000000000000, -0.000000000000000000 ) ) ;
#7128=EDGE_CURVE ( 'NONE', #8282, #7233, #24701, .T. ) ;
#7140=ORIENTED_EDGE ( 'NONE', *, *, #12795, .T. ) ;
#7154=CARTESIAN_POINT ( 'NONE',  ( -2.174791880140518163, 73.99999999999997158, 14.05554496361005334 ) ) ;
#7187=DIRECTION ( 'NONE',  ( 0.000000000000000000, 1.000000000000000000, 0.000000000000000000 ) ) ;
#7197=CARTESIAN_POINT ( 'NONE',  ( 9.270509831248423538, 79.30000000000001137, -12.75976212528059861 ) ) ;
#7209=CARTESIAN_POINT ( 'NONE',  ( 15.00000000000000000, 79.25000000546239676, -1.836970198721029589E-15 ) ) ;
#7214=DIRECTION ( 'NONE',  ( -0.8660254037844410391, 0.4999999999999958367, 0.000000000000000000 ) ) ;
#7221=CARTESIAN_POINT ( 'NONE',  ( 2.688165632520823219E-15, 75.37500000273118417, 14.63369212191046387 ) ) ;
#7233=VERTEX_POINT ( 'NONE', #6010 ) ;
#7243=LINE ( 'NONE', #6906, #30440 ) ;
#7283=DIRECTION ( 'NONE',  ( 0.000000000000000000, 0.000000000000000000, -1.000000000000000000 ) ) ;
#7288=CARTESIAN_POINT ( 'NONE',  ( 2.375766604868044141, 81.44874571845313938, -14.99999999999999822 ) ) ;
#7327=CARTESIAN_POINT ( 'NONE',  ( -14.92155348893272837, 73.99999999999998579, 1.191227978897531958 ) ) ;
#7358=EDGE_CURVE ( 'NONE', #12253, #29760, #3665, .T. ) ;
#7359=FACE_OUTER_BOUND ( 'NONE', #23670, .T. ) ;
#7372=CARTESIAN_POINT ( 'NONE',  ( -12.13525491562421088, 79.80000000000003979, -8.816778784387096835 ) ) ;
#7382=CARTESIAN_POINT ( 'NONE',  ( 13.91746824999999532, 74.47500000273122112, -4.522059556121118540 ) ) ;
#7384=CARTESIAN_POINT ( 'NONE',  ( 15.00000000000000355, 77.15000000546237402, 4.873795443493592394 ) ) ;
#7397=CARTESIAN_POINT ( 'NONE',  ( 13.91746824999999532, 73.97500000273115006, -4.522059556121118540 ) ) ;
#7402=CARTESIAN_POINT ( 'NONE',  ( -8.891200544363830713E-16, 79.49999999999998579, -15.00000000000000000 ) ) ;
#7432=EDGE_CURVE ( 'NONE', #11746, #18278, #8847, .T. ) ;
#7439=VECTOR ( 'NONE', #26733, 1000.000000000000000 ) ;
#7448=ORIENTED_EDGE ( 'NONE', *, *, #9354, .F. ) ;
#7505=CARTESIAN_POINT ( 'NONE',  ( -8.891200544363830713E-16, 77.75000000546235412, -15.00000000000000000 ) ) ;
#7544=CARTESIAN_POINT ( 'NONE',  ( 12.13525491562421088, 76.80000000000003979, 8.816778784387095058 ) ) ;
#7560=ADVANCED_FACE ( 'NONE', ( #7359 ), #8003, .T. ) ;
#7569=CARTESIAN_POINT ( 'NONE',  ( 8.601468415847520532, 74.07500000273121543, 11.83890561707634781 ) ) ;
#7692=FACE_OUTER_BOUND ( 'NONE', #16866, .T. ) ;
#7709=CARTESIAN_POINT ( 'NONE',  ( 4.635254915624209993, 79.65000000546234560, -14.26584774442730463 ) ) ;
#7712=CARTESIAN_POINT ( 'NONE',  ( 12.13525491562421088, 74.80000000000003979, 8.816778784387095058 ) ) ;
#7725=PLANE ( 'NONE',  #6778 ) ;
#7732=CARTESIAN_POINT ( 'NONE',  ( 11.25946833292375793, 78.07500000273121543, -8.180482586598735395 ) ) ;
#7735=CARTESIAN_POINT ( 'NONE',  ( -11.25946833292375793, 79.57500000273121543, 8.180482586598737171 ) ) ;
#7754=CARTESIAN_POINT ( 'NONE',  ( -8.891200544363830713E-16, 75.75000000546238255, -15.00000000000000000 ) ) ;
#7769=ORIENTED_EDGE ( 'NONE', *, *, #1644, .F. ) ;
#7784=ORIENTED_EDGE ( 'NONE', *, *, #10090, .T. ) ;
#7845=AXIS2_PLACEMENT_3D ( 'NONE', #33545, #28231, #5233 ) ;
#7891=CARTESIAN_POINT ( 'NONE',  ( -3.859555026111434639, 74.00000000000001421, -14.20191393030580151 ) ) ;
#7895=ADVANCED_FACE ( 'NONE', ( #26704, #3201 ), #8501, .T. ) ;
#7904=CARTESIAN_POINT ( 'NONE',  ( 12.86449124955741041, 74.00000000000001421, -5.310441354522136947 ) ) ;
#7907=CARTESIAN_POINT ( 'NONE',  ( 13.91746825000000065, 78.27500000273118985, 4.522059556121114987 ) ) ;
#7926=CARTESIAN_POINT ( 'NONE',  ( 8.122944958617804190, 74.00000000000000000, 11.31021757173031972 ) ) ;
#7934=DIRECTION ( 'NONE',  ( -3.169619151431772337E-17, -0.9659258262890680902, -0.2588190451025213501 ) ) ;
#7940=( GEOMETRIC_REPRESENTATION_CONTEXT ( 3 ) GLOBAL_UNCERTAINTY_ASSIGNED_CONTEXT ( ( #21957 ) ) GLOBAL_UNIT_ASSIGNED_CONTEXT ( ( #13404, #23535, #13226 ) ) REPRESENTATION_CONTEXT ( 'NONE', 'WORKASPACE' ) );
#7949=EDGE_CURVE ( 'NONE', #8542, #17164, #15010, .T. ) ;
#7993=EDGE_CURVE ( 'NONE', #25120, #4231, #15506, .T. ) ;
#8003=CYLINDRICAL_SURFACE ( 'NONE', #30195, 15.00000000000000000 ) ;
#8024=CARTESIAN_POINT ( 'NONE',  ( -15.00000000000000000, 70.25000000546238255, 0.000000000000000000 ) ) ;
#8051=CARTESIAN_POINT ( 'NONE',  ( 15.00000000000000355, 72.90000000000001990, 4.873795443493592394 ) ) ;
#8061=CARTESIAN_POINT ( 'NONE',  ( -2.986717648272234182, 74.00000000000000000, -14.37702829354413581 ) ) ;
#8063=DIRECTION ( 'NONE',  ( 1.000000000000000000, 0.000000000000000000, -0.000000000000000000 ) ) ;
#8070=CARTESIAN_POINT ( 'NONE',  ( 0.000000000000000000, 86.00000000000001421, 0.000000000000000000 ) ) ;
#8071=CARTESIAN_POINT ( 'NONE',  ( 11.25946833292375793, 75.67500000273119554, 8.180482586598731842 ) ) ;
#8074=CARTESIAN_POINT ( 'NONE',  ( 13.91746824999999887, 78.37500000273116996, -1.704398294459741270E-15 ) ) ;
#8091=CARTESIAN_POINT ( 'NONE',  ( -4.300734207923755825, 77.77500000273118985, 13.23629886949340673 ) ) ;
#8095=CARTESIAN_POINT ( 'NONE',  ( 12.86449124955741041, 74.00000000000001421, -5.310441354522136947 ) ) ;
#8105=CARTESIAN_POINT ( 'NONE',  ( -1.631291757790872152E-15, 111.9999999999999858, -13.32050807568876927 ) ) ;
#8123=ORIENTED_EDGE ( 'NONE', *, *, #4947, .F. ) ;
#8160=ORIENTED_EDGE ( 'NONE', *, *, #30246, .T. ) ;
#8189=CARTESIAN_POINT ( 'NONE',  ( 12.13525491562420910, 73.45000000546237118, -8.816778784387098611 ) ) ;
#8234=CARTESIAN_POINT ( 'NONE',  ( 13.91746824999999887, 79.87500000273118417, -1.704398294459741270E-15 ) ) ;
#8237=CARTESIAN_POINT ( 'NONE',  ( -4.300734207923755825, 73.77500000273118985, 13.23629886949340673 ) ) ;
#8251=CARTESIAN_POINT ( 'NONE',  ( 8.601468415847520532, 76.07500000273115859, 11.83890561707634781 ) ) ;
#8282=VERTEX_POINT ( 'NONE', #33361 ) ;
#8284=CARTESIAN_POINT ( 'NONE',  ( 4.635254915624212657, 76.59999999999999432, 14.26584774442730286 ) ) ;
#8347=FACE_OUTER_BOUND ( 'NONE', #14708, .T. ) ;
#8352=CARTESIAN_POINT ( 'NONE',  ( 13.91746824999999532, 79.97500000273115006, -4.522059556121118540 ) ) ;
#8379=FACE_OUTER_BOUND ( 'NONE', #24261, .T. ) ;
#8382=CARTESIAN_POINT ( 'NONE',  ( 15.00000000000000000, 73.00000000000001421, -1.836970198721029589E-15 ) ) ;
#8391=CARTESIAN_POINT ( 'NONE',  ( -1.525229598305639200, 73.99999999999998579, -14.55759990445270269 ) ) ;
#8401=CIRCLE ( 'NONE', #728, 15.00000000000000000 ) ;
#8402=CARTESIAN_POINT ( 'NONE',  ( 11.25946833292375793, 76.07500000273120122, -8.180482586598735395 ) ) ;
#8446=CARTESIAN_POINT ( 'NONE',  ( 11.25946833292375793, 80.07500000273121543, -8.180482586598735395 ) ) ;
#8488=CARTESIAN_POINT ( 'NONE',  ( 0.000000000000000000, 74.00000000000001421, 15.00000000000000000 ) ) ;
#8491=CARTESIAN_POINT ( 'NONE',  ( 23.09401076758502569, 96.00000000000002842, -6.857326241137392698E-15 ) ) ;
#8501=PLANE ( 'NONE',  #21463 ) ;
#8502=ORIENTED_EDGE ( 'NONE', *, *, #9354, .T. ) ;
#8512=VECTOR ( 'NONE', #33159, 1000.000000000000000 ) ;
#8524=CARTESIAN_POINT ( 'NONE',  ( 12.13525491562421088, 71.05000000546240813, 8.816778784387095058 ) ) ;
#8535=VECTOR ( 'NONE', #11078, 1000.000000000000000 ) ;
#8542=VERTEX_POINT ( 'NONE', #5819 ) ;
#8547=LINE ( 'NONE', #16454, #23332 ) ;
#8558=( LENGTH_UNIT ( ) NAMED_UNIT ( * ) SI_UNIT ( .MILLI., .METRE. ) );
#8568=( BOUNDED_CURVE ( )  B_SPLINE_CURVE ( 2, ( #17614, #14527, #20194, #4732, #14699, #27910, #28076, #17274, #4565, #32700, #14866, #24818, #30294 ),
 .UNSPECIFIED., .F., .T. ) 
 B_SPLINE_CURVE_WITH_KNOTS ( ( 3, 2, 2, 2, 2, 2, 3 ),
 ( 0.3500000000000000333, 0.3599999999999999867, 0.3800000000000000044, 0.4000000000000000222, 0.4199999999999999845, 0.4400000000000000022, 0.4500000000000000111 ),
 .UNSPECIFIED. ) 
 CURVE ( )  GEOMETRIC_REPRESENTATION_ITEM ( )  RATIONAL_B_SPLINE_CURVE ( ( 0.9755282581475768211, 0.9755282581475768211, 1.000000000000000000, 0.9510565162951535312, 1.000000000000000000, 0.9510565162951535312, 1.000000000000000000, 0.9510565162951535312, 1.000000000000000000, 0.9510565162951535312, 1.000000000000000000, 0.9755282581475768211, 0.9755282581475768211 ) ) 
 REPRESENTATION_ITEM ( '' )  );
#8573=FACE_OUTER_BOUND ( 'NONE', #18017, .T. ) ;
#8577=CARTESIAN_POINT ( 'NONE',  ( -8.601468415847515203, 71.67500000273116711, 11.83890561707634959 ) ) ;
#8590=CARTESIAN_POINT ( 'NONE',  ( -11.25946833292375793, 79.17500000273119554, -8.180482586598733619 ) ) ;
#8605=VERTEX_POINT ( 'NONE', #31725 ) ;
#8606=AXIS2_PLACEMENT_3D ( 'NONE', #12627, #10399, #23275 ) ;
#8618=CARTESIAN_POINT ( 'NONE',  ( 4.300734207923761154, 77.47500000273116427, 13.23629886949340495 ) ) ;
#8627=ORIENTED_EDGE ( 'NONE', *, *, #4965, .T. ) ;
#8630=ORIENTED_EDGE ( 'NONE', *, *, #2230, .F. ) ;
#8638=DIRECTION ( 'NONE',  ( -1.000000000000000000, 0.000000000000000000, 0.000000000000000000 ) ) ;
#8661=CONICAL_SURFACE ( 'NONE', #27847, 14.00000000000000178, 0.2617993877991500740 ) ;
#8686=CARTESIAN_POINT ( 'NONE',  ( 0.000000000000000000, 96.00000000000002842, 0.000000000000000000 ) ) ;
#8690=CARTESIAN_POINT ( 'NONE',  ( 9.270509831248423538, 73.55000000546235128, -12.75976212528059861 ) ) ;
#8742=CARTESIAN_POINT ( 'NONE',  ( 0.000000000000000000, 74.00000000000001421, 0.000000000000000000 ) ) ;
#8748=ORIENTED_EDGE ( 'NONE', *, *, #24249, .T. ) ;
#8755=CARTESIAN_POINT ( 'NONE',  ( 11.25946833292375793, 80.57500000273121543, -8.180482586598735395 ) ) ;
#8764=CARTESIAN_POINT ( 'NONE',  ( -8.960552108402744065E-16, 76.87500000273118417, -14.63369212191046209 ) ) ;
#8779=CARTESIAN_POINT ( 'NONE',  ( 13.91746825000000065, 77.77500000273114722, 4.522059556121114987 ) ) ;
#8783=ORIENTED_EDGE ( 'NONE', *, *, #25934, .F. ) ;
#8807=EDGE_LOOP ( 'NONE', ( #24411, #7448, #8959, #30301 ) ) ;
#8831=ADVANCED_FACE ( 'NONE', ( #29982 ), #26404, .T. ) ;
#8838=CARTESIAN_POINT ( 'NONE',  ( 2.445080149700053643E-15, 74.75000000546239676, 15.00000000000000000 ) ) ;
#8847=CIRCLE ( 'NONE', #5010, 10.64101615137753676 ) ;
#8854=CARTESIAN_POINT ( 'NONE',  ( 4.300734207923761154, 73.47500000273116427, 13.23629886949340495 ) ) ;
#8859=CARTESIAN_POINT ( 'NONE',  ( 8.891200544363830713E-16, 79.75000000546238255, -15.00000000000000000 ) ) ;
#8860=CARTESIAN_POINT ( 'NONE',  ( -4.635254915624208216, 80.39999999999997726, 14.26584774442730463 ) ) ;
#8875=ORIENTED_EDGE ( 'NONE', *, *, #15988, .T. ) ;
#8884=DIRECTION ( 'NONE',  ( -0.000000000000000000, -1.000000000000000000, -0.000000000000000000 ) ) ;
#8907=CARTESIAN_POINT ( 'NONE',  ( 13.91746824999999887, 72.37500000273116996, -1.704398294459741270E-15 ) ) ;
#8923=CARTESIAN_POINT ( 'NONE',  ( -13.91746824999999887, 73.37500000273116996, 0.000000000000000000 ) ) ;
#8935=CARTESIAN_POINT ( 'NONE',  ( 8.601468415847520532, 80.07500000273121543, 11.83890561707634603 ) ) ;
#8944=CARTESIAN_POINT ( 'NONE',  ( -11.54700538379251817, 96.00000000000002842, 19.99999999999999645 ) ) ;
#8952=CARTESIAN_POINT ( 'NONE',  ( -4.300734207923759378, 80.47500000273116427, -13.23629886949340495 ) ) ;
#8959=ORIENTED_EDGE ( 'NONE', *, *, #20203, .T. ) ;
#9023=CARTESIAN_POINT ( 'NONE',  ( -8.601468415847518756, 76.57500000273120122, -11.83890561707634781 ) ) ;
#9074=DIRECTION ( 'NONE',  ( -0.000000000000000000, -1.000000000000000000, -0.000000000000000000 ) ) ;
#9084=VERTEX_POINT ( 'NONE', #33409 ) ;
#9092=CARTESIAN_POINT ( 'NONE',  ( 13.91746824999999887, 72.37500000273116996, -1.704398294459741270E-15 ) ) ;
#9102=CARTESIAN_POINT ( 'NONE',  ( -13.91746824999999532, 79.47500000273116427, 4.522059556121122093 ) ) ;
#9105=EDGE_LOOP ( 'NONE', ( #28929, #15140, #32299, #9590 ) ) ;
#9116=CARTESIAN_POINT ( 'NONE',  ( -13.91746824999999532, 76.77500000273118985, -4.522059556121115875 ) ) ;
#9126=ORIENTED_EDGE ( 'NONE', *, *, #24474, .F. ) ;
#9127=EDGE_LOOP ( 'NONE', ( #8502, #3832 ) ) ;
#9144=FACE_OUTER_BOUND ( 'NONE', #17034, .T. ) ;
#9146=ADVANCED_FACE ( 'NONE', ( #20383, #9730 ), #17636, .F. ) ;
#9153=CARTESIAN_POINT ( 'NONE',  ( -11.25946833292375793, 80.67500000273119554, -8.180482586598733619 ) ) ;
#9156=SURFACE_SIDE_STYLE ('',( #22214 ) ) ;
#9164=ORIENTED_EDGE ( 'NONE', *, *, #11001, .T. ) ;
#9166=CARTESIAN_POINT ( 'NONE',  ( -23.09401076758502924, 86.00000000000001421, 5.354274672883389237E-15 ) ) ;
#9185=CARTESIAN_POINT ( 'NONE',  ( -4.300734207923759378, 72.47500000273116427, -13.23629886949340495 ) ) ;
#9215=CARTESIAN_POINT ( 'NONE',  ( -15.00000000000000000, 74.00000000000001421, 0.000000000000000000 ) ) ;
#9244=EDGE_CURVE ( 'NONE', #29890, #22018, #22779, .T. ) ;
#9254=CARTESIAN_POINT ( 'NONE',  ( -15.00000000000000000, 80.10000000000003695, 4.873795443493597723 ) ) ;
#9266=CARTESIAN_POINT ( 'NONE',  ( -12.13525491562421088, 80.05000000546236549, -8.816778784387096835 ) ) ;
#9278=CARTESIAN_POINT ( 'NONE',  ( 2.688165632520823219E-15, 71.37500000273119838, 14.63369212191046387 ) ) ;
#9306=DIRECTION ( 'NONE',  ( -0.000000000000000000, 1.000000000000000000, -0.000000000000000000 ) ) ;
#9324=PRODUCT_DEFINITION_FORMATION_WITH_SPECIFIED_SOURCE ( 'ANY', '', #12, .NOT_KNOWN. ) ;
#9349=CARTESIAN_POINT ( 'NONE',  ( -13.91746824999999887, 76.87500000273116996, 0.000000000000000000 ) ) ;
#9354=EDGE_CURVE ( 'NONE', #18278, #11746, #13813, .T. ) ;
#9381=CARTESIAN_POINT ( 'NONE',  ( -11.54700538379251995, 86.00000000000001421, -19.99999999999999645 ) ) ;
#9414=VERTEX_POINT ( 'NONE', #1105 ) ;
#9422=CARTESIAN_POINT ( 'NONE',  ( 11.25946833292375793, 74.17500000273119554, 8.180482586598731842 ) ) ;
#9433=CARTESIAN_POINT ( 'NONE',  ( 11.25946833292375793, 78.57500000273121543, -8.180482586598735395 ) ) ;
#9435=CARTESIAN_POINT ( 'NONE',  ( -9.270509831248421762, 78.55000000546236549, 12.75976212528060039 ) ) ;
#9442=AXIS2_PLACEMENT_3D ( 'NONE', #20759, #5632, #12848 ) ;
#9451=CARTESIAN_POINT ( 'NONE',  ( 13.91746824999999532, 71.97500000273117848, -4.522059556121118540 ) ) ;
#9461=VERTEX_POINT ( 'NONE', #10220 ) ;
#9481=DIRECTION ( 'NONE',  ( -0.000000000000000000, 1.000000000000000000, -0.000000000000000000 ) ) ;
#9500=CARTESIAN_POINT ( 'NONE',  ( 0.000000000000000000, 74.00000000000001421, 0.000000000000000000 ) ) ;
#9562=CARTESIAN_POINT ( 'NONE',  ( -4.491574677915616043, 74.00000000000000000, 13.59926041343836012 ) ) ;
#9584=CARTESIAN_POINT ( 'NONE',  ( 11.54700538379251107, 96.00000000000002842, -19.99999999999999645 ) ) ;
#9590=ORIENTED_EDGE ( 'NONE', *, *, #30738, .T. ) ;
#9603=CARTESIAN_POINT ( 'NONE',  ( -15.00000000000000000, 81.89999999999997726, -4.873795443493594171 ) ) ;
#9614=CARTESIAN_POINT ( 'NONE',  ( 4.635254915624209993, 79.65000000546234560, -14.26584774442730463 ) ) ;
#9627=CARTESIAN_POINT ( 'NONE',  ( -13.91746824999999532, 74.97500000273117848, 4.522059556121122093 ) ) ;
#9632=CARTESIAN_POINT ( 'NONE',  ( 4.635254915624209993, 79.39999999999997726, -14.26584774442730463 ) ) ;
#9691=DIRECTION ( 'NONE',  ( 0.000000000000000000, -1.000000000000000000, 0.000000000000000000 ) ) ;
#9730=FACE_OUTER_BOUND ( 'NONE', #27660, .T. ) ;
#9752=CARTESIAN_POINT ( 'NONE',  ( -2.375766604868044585, 78.69874572391550771, 14.99999999999999822 ) ) ;
#9764=CARTESIAN_POINT ( 'NONE',  ( 0.000000000000000000, 102.0000000000000284, 0.000000000000000000 ) ) ;
#9771=CARTESIAN_POINT ( 'NONE',  ( 15.00000000000000355, 79.15000000546235981, 4.873795443493592394 ) ) ;
#9775=CARTESIAN_POINT ( 'NONE',  ( 2.897257156509938333E-15, 78.49999999999994316, 15.77193336357400710 ) ) ;
#9789=CARTESIAN_POINT ( 'NONE',  ( -12.13525491562420910, 78.45000000546237118, 8.816778784387098611 ) ) ;
#9790=EDGE_CURVE ( 'NONE', #30951, #6130, #17044, .T. ) ;
#9804=CARTESIAN_POINT ( 'NONE',  ( -13.91746824999999532, 72.77500000273120406, -4.522059556121115875 ) ) ;
#9808=DIRECTION ( 'NONE',  ( -0.5000000000000000000, 0.000000000000000000, -0.8660254037844385966 ) ) ;
#9849=PLANE ( 'NONE',  #33079 ) ;
#9875=CARTESIAN_POINT ( 'NONE',  ( 2.688165632520823219E-15, 71.37500000273119838, 14.63369212191046387 ) ) ;
#9951=CARTESIAN_POINT ( 'NONE',  ( 9.270509831248423538, 77.30000000000001137, -12.75976212528059861 ) ) ;
#9961=CARTESIAN_POINT ( 'NONE',  ( 5.348221797398307942, 74.00000000000001421, 12.84883053416113974 ) ) ;
#9963=CARTESIAN_POINT ( 'NONE',  ( -15.00000000000000000, 74.15000000546240244, -4.873795443493594171 ) ) ;
#9976=CARTESIAN_POINT ( 'NONE',  ( -11.25946833292375793, 74.67500000273119554, -8.180482586598733619 ) ) ;
#10028=PLANE ( 'NONE',  #10641 ) ;
#10090=EDGE_CURVE ( 'NONE', #11746, #25891, #7243, .T. ) ;
#10122=CARTESIAN_POINT ( 'NONE',  ( 2.375766604868043697, 78.80125428700924317, 15.00000000000000178 ) ) ;
#10125=CARTESIAN_POINT ( 'NONE',  ( -15.00000000000000000, 80.00000000000001421, 0.000000000000000000 ) ) ;
#10146=CARTESIAN_POINT ( 'NONE',  ( -4.635254915624211769, 81.60000000000000853, -14.26584774442730286 ) ) ;
#10150=CARTESIAN_POINT ( 'NONE',  ( 11.25946833292375793, 78.17500000273119554, 8.180482586598731842 ) ) ;
#10220=CARTESIAN_POINT ( 'NONE',  ( 1.469576158976824144E-15, 102.0000000000000284, 12.00000000000000178 ) ) ;
#10230=CARTESIAN_POINT ( 'NONE',  ( 2.445080149700053643E-15, 74.49999999999998579, 15.00000000000000000 ) ) ;
#10275=DIRECTION ( 'NONE',  ( 0.000000000000000000, 0.000000000000000000, 1.000000000000000000 ) ) ;
#10298=CARTESIAN_POINT ( 'NONE',  ( -9.657523855033125146E-16, 75.50000000000001421, -15.77193336357400710 ) ) ;
#10301=DIRECTION ( 'NONE',  ( -0.000000000000000000, -1.000000000000000000, -0.000000000000000000 ) ) ;
#10317=CARTESIAN_POINT ( 'NONE',  ( 4.300734207923757602, 74.27500000273118985, -13.23629886949340673 ) ) ;
#10322=CARTESIAN_POINT ( 'NONE',  ( 13.91746824999999887, 76.37500000273116996, -1.704398294459741270E-15 ) ) ;
#10351=DIRECTION ( 'NONE',  ( -0.000000000000000000, -1.000000000000000000, -0.000000000000000000 ) ) ;
#10367=EDGE_LOOP ( 'NONE', ( #16211, #11377 ) ) ;
#10399=DIRECTION ( 'NONE',  ( -0.000000000000000000, -1.000000000000000000, -0.000000000000000000 ) ) ;
#10457=VERTEX_POINT ( 'NONE', #29197 ) ;
#10462=CARTESIAN_POINT ( 'NONE',  ( -9.270509831248425314, 77.70000000000000284, -12.75976212528059861 ) ) ;
#10483=CARTESIAN_POINT ( 'NONE',  ( -13.91746824999999887, 78.87500000273118417, 0.000000000000000000 ) ) ;
#10486=CARTESIAN_POINT ( 'NONE',  ( 4.300734207923757602, 74.77500000273118985, -13.23629886949340673 ) ) ;
#10506=CARTESIAN_POINT ( 'NONE',  ( 12.07957071404696592, 74.00000000000001421, 6.971801377361973806 ) ) ;
#10515=LINE ( 'NONE', #28866, #5104 ) ;
#10591=AXIS2_PLACEMENT_3D ( 'NONE', #18177, #4775, #17656 ) ;
#10604=CARTESIAN_POINT ( 'NONE',  ( 2.897257156509938333E-15, 70.75000000546238255, 15.77193336357400710 ) ) ;
#10609=DIRECTION ( 'NONE',  ( 0.000000000000000000, 0.000000000000000000, 1.000000000000000000 ) ) ;
#10641=AXIS2_PLACEMENT_3D ( 'NONE', #9500, #20326, #25471 ) ;
#10642=CARTESIAN_POINT ( 'NONE',  ( 12.86449124955741041, 74.00000000000001421, -5.310441354522136947 ) ) ;
#10653=CARTESIAN_POINT ( 'NONE',  ( 2.688165632520823219E-15, 79.37500000273118417, 14.63369212191046209 ) ) ;
#10656=CARTESIAN_POINT ( 'NONE',  ( -4.300734207923755825, 77.77500000273118985, 13.23629886949340673 ) ) ;
#10671=CARTESIAN_POINT ( 'NONE',  ( -8.960552108402742093E-16, 76.87500000273118417, -14.63369212191046387 ) ) ;
#10674=CARTESIAN_POINT ( 'NONE',  ( 6.189173980287828059, 74.00000000000002842, 12.49879098907252128 ) ) ;
#10703=EDGE_CURVE ( 'NONE', #4231, #17758, #14024, .T. ) ;
#10753=EDGE_LOOP ( 'NONE', ( #26841, #32316, #33359, #26027 ) ) ;
#10765=B_SPLINE_CURVE_WITH_KNOTS ( 'NONE', 3,
 ( #8095, #26292, #10845, #24059, #26460, #18, #26794, #23720, #16338, #20984, #527, #29190, #10506, #3286, #18582, #18913, #13754, #23890, #7926, #13595, #10674, #24225 ),
 .UNSPECIFIED., .F., .F.,
 ( 4, 2, 2, 2, 2, 2, 2, 2, 2, 2, 4 ),
 ( 2.442512830937285584E-16, 0.002730916255965320019, 0.005461832511930396310, 0.008192748767895472600, 0.009558206895878010312, 0.01092366502386054629, 0.01365458127982561651, 0.01638549753579068499, 0.01775095566377321576, 0.01911641379175575001, 0.02184733004772081155 ),
 .UNSPECIFIED. ) ;
#10775=CARTESIAN_POINT ( 'NONE',  ( 15.00000000000000000, 73.25000000546239676, -1.836970198721029589E-15 ) ) ;
#10802=CARTESIAN_POINT ( 'NONE',  ( 12.13525491562421088, 72.80000000000002558, 8.816778784387095058 ) ) ;
#10812=CARTESIAN_POINT ( 'NONE',  ( -3.278034869283648511, 74.00000000000002842, -14.32477225908124829 ) ) ;
#10823=CARTESIAN_POINT ( 'NONE',  ( -4.300734207923759378, 78.47500000273116427, -13.23629886949340495 ) ) ;
#10826=CARTESIAN_POINT ( 'NONE',  ( 13.91746824999999887, 74.37500000273116996, -1.704398294459741270E-15 ) ) ;
#10838=CARTESIAN_POINT ( 'NONE',  ( -11.54700538379251995, 96.00000000000002842, -19.99999999999999645 ) ) ;
#10841=CARTESIAN_POINT ( 'NONE',  ( 13.91746824999999887, 76.37500000273116996, -1.704398294459741270E-15 ) ) ;
#10845=CARTESIAN_POINT ( 'NONE',  ( 13.47594703999181043, 74.00000000000000000, -3.594779225894267682 ) ) ;
#10877=CARTESIAN_POINT ( 'NONE',  ( 9.270509831248425314, 76.70000000000001705, 12.75976212528059683 ) ) ;
#10880=ORIENTED_EDGE ( 'NONE', *, *, #7358, .T. ) ;
#10941=CARTESIAN_POINT ( 'NONE',  ( -4.635254915624211769, 71.85000000546237686, -14.26584774442730286 ) ) ;
#10992=CARTESIAN_POINT ( 'NONE',  ( 8.601468415847520532, 77.57500000273117280, 11.83890561707634603 ) ) ;
#11001=EDGE_CURVE ( 'NONE', #220, #13542, #16672, .T. ) ;
#11010=CARTESIAN_POINT ( 'NONE',  ( -11.25946833292375793, 81.17500000273119554, -8.180482586598733619 ) ) ;
#11014=DIRECTION ( 'NONE',  ( 0.000000000000000000, 0.000000000000000000, -1.000000000000000000 ) ) ;
#11037=CARTESIAN_POINT ( 'NONE',  ( -13.91746824999999532, 78.77500000273117564, -4.522059556121115875 ) ) ;
#11060=CARTESIAN_POINT ( 'NONE',  ( -15.00000000000000000, 80.25000000546239676, 0.000000000000000000 ) ) ;
#11078=DIRECTION ( 'NONE',  ( 0.000000000000000000, -0.9659258262890680902, 0.2588190451025213501 ) ) ;
#11112=CARTESIAN_POINT ( 'NONE',  ( -8.601468415847518756, 80.57500000273118701, -11.83890561707634781 ) ) ;
#11123=CARTESIAN_POINT ( 'NONE',  ( 2.445080149700053643E-15, 74.75000000546239676, 15.00000000000000000 ) ) ;
#11140=CARTESIAN_POINT ( 'NONE',  ( 15.00000000000000000, 73.10000000000000853, -4.873795443493596835 ) ) ;
#11142=CARTESIAN_POINT ( 'NONE',  ( 0.000000000000000000, 122.0000000000000000, 0.000000000000000000 ) ) ;
#11163=CARTESIAN_POINT ( 'NONE',  ( -11.25946833292375793, 73.57500000273120122, 8.180482586598737171 ) ) ;
#11166=ORIENTED_EDGE ( 'NONE', *, *, #17545, .F. ) ;
#11177=CARTESIAN_POINT ( 'NONE',  ( -8.960552108402742093E-16, 80.87500000273116996, -14.63369212191046387 ) ) ;
#11226=LINE ( 'NONE', #21702, #19944 ) ;
#11228=VERTEX_POINT ( 'NONE', #25057 ) ;
#11256=ORIENTED_EDGE ( 'NONE', *, *, #23684, .F. ) ;
#11266=CARTESIAN_POINT ( 'NONE',  ( 4.635254915624212657, 76.85000000546237686, 14.26584774442730286 ) ) ;
#11275=CARTESIAN_POINT ( 'NONE',  ( 13.91746824999999887, 79.87500000273118417, -1.704398294459741270E-15 ) ) ;
#11323=CARTESIAN_POINT ( 'NONE',  ( 8.601468415847516980, 72.67500000273120975, -11.83890561707634781 ) ) ;
#11327=VECTOR ( 'NONE', #7214, 1000.000000000000114 ) ;
#11338=CARTESIAN_POINT ( 'NONE',  ( 13.91746825000000065, 80.27500000273120406, 4.522059556121114987 ) ) ;
#11347=CARTESIAN_POINT ( 'NONE',  ( 11.25946833292375793, 80.17500000273119554, 8.180482586598731842 ) ) ;
#11365=CARTESIAN_POINT ( 'NONE',  ( -13.91746824999999887, 80.87500000273118417, 0.000000000000000000 ) ) ;
#11377=ORIENTED_EDGE ( 'NONE', *, *, #11586, .T. ) ;
#11389=ORIENTED_EDGE ( 'NONE', *, *, #30246, .F. ) ;
#11419=CARTESIAN_POINT ( 'NONE',  ( 9.270509831248425314, 74.95000000546237118, 12.75976212528059683 ) ) ;
#11433=CARTESIAN_POINT ( 'NONE',  ( 13.91746824999999887, 75.87500000273116996, -1.704398294459741270E-15 ) ) ;
#11436=DIRECTION ( 'NONE',  ( 0.000000000000000000, 0.000000000000000000, 1.000000000000000000 ) ) ;
#11439=CARTESIAN_POINT ( 'NONE',  ( -15.00000000000000000, 80.00000000000001421, 0.000000000000000000 ) ) ;
#11487=CARTESIAN_POINT ( 'NONE',  ( -11.25946833292375793, 71.57500000273120122, 8.180482586598737171 ) ) ;
#11499=CARTESIAN_POINT ( 'NONE',  ( -13.91746824999999887, 71.37500000273116996, 0.000000000000000000 ) ) ;
#11508=CARTESIAN_POINT ( 'NONE',  ( -4.300734207923759378, 78.97500000273122112, -13.23629886949340495 ) ) ;
#11523=CARTESIAN_POINT ( 'NONE',  ( 11.25946833292375793, 77.67500000273119554, 8.180482586598731842 ) ) ;
#11551=ORIENTED_EDGE ( 'NONE', *, *, #22368, .T. ) ;
#11562=CARTESIAN_POINT ( 'NONE',  ( -15.00000000000000000, 82.00000000000001421, 0.000000000000000000 ) ) ;
#11566=VECTOR ( 'NONE', #27370, 1000.000000000000227 ) ;
#11579=ORIENTED_EDGE ( 'NONE', *, *, #22904, .F. ) ;
#11586=EDGE_CURVE ( 'NONE', #4172, #9084, #26643, .T. ) ;
#11598=CARTESIAN_POINT ( 'NONE',  ( -4.300734207923759378, 74.47500000273116427, -13.23629886949340495 ) ) ;
#11632=PRESENTATION_STYLE_ASSIGNMENT (( #14384 ) ) ;
#11645=UNCERTAINTY_MEASURE_WITH_UNIT (LENGTH_MEASURE( 1.000000000000000082E-05 ), #8558, 'distance_accuracy_value', 'NONE');
#11653=AXIS2_PLACEMENT_3D ( 'NONE', #335, #13899, #16315 ) ;
#11668=CARTESIAN_POINT ( 'NONE',  ( 2.897257156509938333E-15, 80.50000000000002842, 15.77193336357400710 ) ) ;
#11677=CARTESIAN_POINT ( 'NONE',  ( 4.300734207923761154, 79.97500000273122112, 13.23629886949340495 ) ) ;
#11683=CYLINDRICAL_SURFACE ( 'NONE', #26133, 15.00000000000000000 ) ;
#11695=ORIENTED_EDGE ( 'NONE', *, *, #2230, .T. ) ;
#11700=CIRCLE ( 'NONE', #187, 12.00000000000000178 ) ;
#11746=VERTEX_POINT ( 'NONE', #33063 ) ;
#11749=CARTESIAN_POINT ( 'NONE',  ( -15.00000000000000000, 75.89999999999996305, -4.873795443493594171 ) ) ;
#11764=CARTESIAN_POINT ( 'NONE',  ( 13.91746825000000065, 73.77500000273116143, 4.522059556121114987 ) ) ;
#11798=CARTESIAN_POINT ( 'NONE',  ( -14.60862552821003213, 74.00000000000002842, 2.946899241987215756 ) ) ;
#11803=( NAMED_UNIT ( * ) PLANE_ANGLE_UNIT ( ) SI_UNIT ( $, .RADIAN. ) );
#11809=VECTOR ( 'NONE', #865, 1000.000000000000114 ) ;
#11837=CARTESIAN_POINT ( 'NONE',  ( -8.601468415847515203, 71.67500000273116711, 11.83890561707634959 ) ) ;
#11846=CARTESIAN_POINT ( 'NONE',  ( 2.688165632520823219E-15, 79.87500000273115575, 14.63369212191046209 ) ) ;
#11848=CARTESIAN_POINT ( 'NONE',  ( 2.897257156509938333E-15, 76.75000000546238255, 15.77193336357400710 ) ) ;
#11861=CARTESIAN_POINT ( 'NONE',  ( -13.91746824999999532, 70.97500000273119269, 4.522059556121122093 ) ) ;
#11895=FACE_OUTER_BOUND ( 'NONE', #32462, .T. ) ;
#11914=AXIS2_PLACEMENT_3D ( 'NONE', #26073, #13375, #18533 ) ;
#11937=CARTESIAN_POINT ( 'NONE',  ( 8.601468415847520532, 73.57500000273117280, 11.83890561707634781 ) ) ;
#11964=CARTESIAN_POINT ( 'NONE',  ( 2.532662468604912398, 74.00000000000004263, 13.81508367526550884 ) ) ;
#11973=CARTESIAN_POINT ( 'NONE',  ( 2.445080149700053643E-15, 76.50000000000001421, 15.00000000000000000 ) ) ;
#11984=CARTESIAN_POINT ( 'NONE',  ( -9.270509831248423538, 77.95000000546239960, -12.75976212528059861 ) ) ;
#12004=CARTESIAN_POINT ( 'NONE',  ( 8.601468415847516980, 74.67500000273120975, -11.83890561707634781 ) ) ;
#12015=CARTESIAN_POINT ( 'NONE',  ( 13.91746824999999887, 76.37500000273116996, -1.704398294459741270E-15 ) ) ;
#12017=CARTESIAN_POINT ( 'NONE',  ( 15.00000000000000000, 77.35000000546234844, -4.873795443493596835 ) ) ;
#12030=CARTESIAN_POINT ( 'NONE',  ( 13.91746824999999887, 80.37500000273118417, -1.704398294459741270E-15 ) ) ;
#12032=CARTESIAN_POINT ( 'NONE',  ( 4.635254915624212657, 78.60000000000000853, 14.26584774442730286 ) ) ;
#12045=APPLICATION_CONTEXT ( 'automotive_design' ) ;
#12060=LINE ( 'NONE', #27859, #24943 ) ;
#12086=CARTESIAN_POINT ( 'NONE',  ( -9.270509831248419985, 76.30000000000003979, 12.75976212528060039 ) ) ;
#12102=CARTESIAN_POINT ( 'NONE',  ( 8.601468415847520532, 75.57500000273117280, 11.83890561707634781 ) ) ;
#12131=CARTESIAN_POINT ( 'NONE',  ( -6.433434964406110623, 74.00000000000001421, 12.87341652790383861 ) ) ;
#12139=LINE ( 'NONE', #33418, #19801 ) ;
#12152=CARTESIAN_POINT ( 'NONE',  ( -15.00000000000000000, 78.35000000546237686, 4.873795443493597723 ) ) ;
#12176=CARTESIAN_POINT ( 'NONE',  ( 8.601468415847516980, 72.67500000273120975, -11.83890561707634781 ) ) ;
#12188=CARTESIAN_POINT ( 'NONE',  ( 9.270509831248423538, 79.55000000546240813, -12.75976212528059861 ) ) ;
#12202=CARTESIAN_POINT ( 'NONE',  ( 4.300734207923757602, 72.27500000273117564, -13.23629886949340673 ) ) ;
#12204=CARTESIAN_POINT ( 'NONE',  ( 11.54700538379251817, 96.00000000000002842, 19.99999999999999645 ) ) ;
#12233=CARTESIAN_POINT ( 'NONE',  ( 1.469576158976824144E-15, 96.00000000000002842, 12.00000000000000000 ) ) ;
#12253=VERTEX_POINT ( 'NONE', #196 ) ;
#12270=CARTESIAN_POINT ( 'NONE',  ( 0.000000000000000000, 96.00000000000002842, 0.000000000000000000 ) ) ;
#12287=COLOUR_RGB ( '', 0.40784314, 0.44705882, 0.49803922) ;
#12299=DIRECTION ( 'NONE',  ( 0.000000000000000000, 0.000000000000000000, 1.000000000000000000 ) ) ;
#12308=CARTESIAN_POINT ( 'NONE',  ( -10.13840065261075551, 73.99999999999994316, 10.46602128917086993 ) ) ;
#12348=CARTESIAN_POINT ( 'NONE',  ( -4.223320258572821363E-15, 78.75000000546236834, 15.00000000000000355 ) ) ;
#12351=CARTESIAN_POINT ( 'NONE',  ( -4.635254915624211769, 77.60000000000000853, -14.26584774442730286 ) ) ;
#12358=EDGE_CURVE ( 'NONE', #30053, #4440, #20994, .T. ) ;
#12363=CARTESIAN_POINT ( 'NONE',  ( -15.00000000000000000, 78.25000000546239676, 0.000000000000000000 ) ) ;
#12376=CARTESIAN_POINT ( 'NONE',  ( -4.300734207923759378, 72.47500000273116427, -13.23629886949340495 ) ) ;
#12433=CIRCLE ( 'NONE', #30490, 12.00000000000000000 ) ;
#12446=CARTESIAN_POINT ( 'NONE',  ( 4.635254915624209993, 81.39999999999997726, -14.26584774442730463 ) ) ;
#12458=DIRECTION ( 'NONE',  ( -0.000000000000000000, 1.000000000000000000, -0.000000000000000000 ) ) ;
#12513=ORIENTED_EDGE ( 'NONE', *, *, #28656, .T. ) ;
#12525=CARTESIAN_POINT ( 'NONE',  ( -12.13525491562421088, 75.80000000000003979, -8.816778784387096835 ) ) ;
#12537=CARTESIAN_POINT ( 'NONE',  ( -4.635254915624208216, 74.65000000546240244, 14.26584774442730463 ) ) ;
#12550=CARTESIAN_POINT ( 'NONE',  ( 4.300734207923761154, 71.47500000273116427, 13.23629886949340495 ) ) ;
#12555=FACE_OUTER_BOUND ( 'NONE', #26279, .T. ) ;
#12595=ORIENTED_EDGE ( 'NONE', *, *, #26240, .F. ) ;
#12627=CARTESIAN_POINT ( 'NONE',  ( 0.000000000000000000, 102.0000000000000284, 0.000000000000000000 ) ) ;
#12658=DIRECTION ( 'NONE',  ( 1.000000000000000000, 0.000000000000000000, 0.000000000000000000 ) ) ;
#12686=ORIENTED_EDGE ( 'NONE', *, *, #30831, .T. ) ;
#12694=CARTESIAN_POINT ( 'NONE',  ( -9.657523855033125146E-16, 79.49999999999998579, -15.77193336357400710 ) ) ;
#12704=CARTESIAN_POINT ( 'NONE',  ( 11.25946833292375793, 74.17500000273119554, 8.180482586598731842 ) ) ;
#12706=CARTESIAN_POINT ( 'NONE',  ( -12.13525491562421088, 72.05000000546240813, -8.816778784387096835 ) ) ;
#12719=CARTESIAN_POINT ( 'NONE',  ( 11.25946833292375793, 74.57500000273120122, -8.180482586598735395 ) ) ;
#12722=CARTESIAN_POINT ( 'NONE',  ( 0.000000000000000000, 111.9999999999999858, 13.32050807568876927 ) ) ;
#12795=EDGE_CURVE ( 'NONE', #6130, #18703, #23866, .T. ) ;
#12797=CARTESIAN_POINT ( 'NONE',  ( -13.91746824999999532, 70.97500000273119269, 4.522059556121122093 ) ) ;
#12803=CARTESIAN_POINT ( 'NONE',  ( -10.58590195883389207, 74.00000000000001421, -10.62726115788808201 ) ) ;
#12843=DIRECTION ( 'NONE',  ( -0.000000000000000000, -1.000000000000000000, -0.000000000000000000 ) ) ;
#12848=DIRECTION ( 'NONE',  ( 0.000000000000000000, 0.000000000000000000, 1.000000000000000000 ) ) ;
#12865=CARTESIAN_POINT ( 'NONE',  ( -4.635254915624208216, 78.39999999999996305, 14.26584774442730463 ) ) ;
#12886=CARTESIAN_POINT ( 'NONE',  ( -13.91746824999999532, 74.97500000273119269, 4.522059556121122093 ) ) ;
#12890=CARTESIAN_POINT ( 'NONE',  ( -11.25946833292375793, 75.17500000273119554, -8.180482586598733619 ) ) ;
#12893=DIRECTION ( 'NONE',  ( 0.000000000000000000, -0.9659258262890680902, 0.2588190451025213501 ) ) ;
#12949=VECTOR ( 'NONE', #13256, 1000.000000000000000 ) ;
#12959=FACE_OUTER_BOUND ( 'NONE', #16536, .T. ) ;
#12967=CARTESIAN_POINT ( 'NONE',  ( 13.91746825000000065, 71.77500000273117564, 4.522059556121114987 ) ) ;
#13012=AXIS2_PLACEMENT_3D ( 'NONE', #31476, #2820, #23763 ) ;
#13014=FACE_OUTER_BOUND ( 'NONE', #26156, .T. ) ;
#13035=ADVANCED_FACE ( 'NONE', ( #29999 ), #6503, .T. ) ;
#13039=CARTESIAN_POINT ( 'NONE',  ( 4.635254915624209993, 79.39999999999997726, -14.26584774442730463 ) ) ;
#13057=CARTESIAN_POINT ( 'NONE',  ( -11.25946833292375793, 74.67500000273119554, -8.180482586598733619 ) ) ;
#13060=CARTESIAN_POINT ( 'NONE',  ( -8.960552108402742093E-16, 74.87500000273119838, -14.63369212191046387 ) ) ;
#13191=EDGE_LOOP ( 'NONE', ( #24396, #2203, #30254, #20076, #25128, #27704 ) ) ;
#13210=CARTESIAN_POINT ( 'NONE',  ( 1.425975843264271514, 74.00000000000001421, -14.45395831230864481 ) ) ;
#13222=CARTESIAN_POINT ( 'NONE',  ( 13.91746824999999532, 77.97500000273122112, -4.522059556121118540 ) ) ;
#13225=CARTESIAN_POINT ( 'NONE',  ( 13.91746824999999532, 76.47500000273120691, -4.522059556121118540 ) ) ;
#13226=( NAMED_UNIT ( * ) SI_UNIT ( $, .STERADIAN. ) SOLID_ANGLE_UNIT ( ) );
#13241=CARTESIAN_POINT ( 'NONE',  ( -8.601468415847518756, 77.07500000273117280, -11.83890561707634781 ) ) ;
#13242=AXIS2_PLACEMENT_3D ( 'NONE', #22366, #33337, #29910 ) ;
#13256=DIRECTION ( 'NONE',  ( 1.000000000000000000, 0.000000000000000000, 0.000000000000000000 ) ) ;
#13257=CARTESIAN_POINT ( 'NONE',  ( 0.000000000000000000, 86.00000000000001421, 0.000000000000000000 ) ) ;
#13277=CARTESIAN_POINT ( 'NONE',  ( 2.375766604868043252, 77.44874571845312516, -14.99999999999999822 ) ) ;
#13348=CARTESIAN_POINT ( 'NONE',  ( 9.270509831248423538, 71.55000000546236549, -12.75976212528059861 ) ) ;
#13357=DIRECTION ( 'NONE',  ( 0.000000000000000000, 0.000000000000000000, 1.000000000000000000 ) ) ;
#13359=CARTESIAN_POINT ( 'NONE',  ( 0.000000000000000000, 74.00000000000001421, -9.000000000000001776 ) ) ;
#13375=DIRECTION ( 'NONE',  ( 0.000000000000000000, 0.000000000000000000, -1.000000000000000000 ) ) ;
#13388=CARTESIAN_POINT ( 'NONE',  ( 3.164787637625844585, 74.00000000000002842, -14.10554145339599152 ) ) ;
#13400=CARTESIAN_POINT ( 'NONE',  ( -4.300734207923755825, 77.27500000273118985, 13.23629886949340673 ) ) ;
#13403=CARTESIAN_POINT ( 'NONE',  ( 13.91746824999999532, 78.47500000273120691, -4.522059556121118540 ) ) ;
#13404=( LENGTH_UNIT ( ) NAMED_UNIT ( * ) SI_UNIT ( .MILLI., .METRE. ) );
#13432=LINE ( 'NONE', #23900, #22083 ) ;
#13453=CARTESIAN_POINT ( 'NONE',  ( 12.13525491562421088, 76.80000000000003979, 8.816778784387095058 ) ) ;
#13457=ORIENTED_EDGE ( 'NONE', *, *, #17205, .T. ) ;
#13462=ORIENTED_EDGE ( 'NONE', *, *, #27079, .F. ) ;
#13503=ORIENTED_EDGE ( 'NONE', *, *, #11001, .F. ) ;
#13518=DIRECTION ( 'NONE',  ( -0.000000000000000000, 1.000000000000000000, -0.000000000000000000 ) ) ;
#13524=CARTESIAN_POINT ( 'NONE',  ( 15.00000000000000355, 73.15000000546237402, 4.873795443493592394 ) ) ;
#13527=CARTESIAN_POINT ( 'NONE',  ( 1.836970198721029589E-15, 74.00000000000001421, -15.00000000000000000 ) ) ;
#13529=CARTESIAN_POINT ( 'NONE',  ( -2.375766604868044141, 79.80125428700922896, -14.99999999999999822 ) ) ;
#13542=VERTEX_POINT ( 'NONE', #28327 ) ;
#13551=CARTESIAN_POINT ( 'NONE',  ( 4.635254915624212657, 72.59999999999999432, 14.26584774442730286 ) ) ;
#13563=CARTESIAN_POINT ( 'NONE',  ( -4.150128892133675862, 74.00000000000002842, -14.13113817901305680 ) ) ;
#13574=ADVANCED_FACE ( 'NONE', ( #8573 ), #19220, .T. ) ;
#13575=CARTESIAN_POINT ( 'NONE',  ( -13.91746824999999887, 74.87500000273116996, 0.000000000000000000 ) ) ;
#13578=FACE_OUTER_BOUND ( 'NONE', #17581, .T. ) ;
#13591=CARTESIAN_POINT ( 'NONE',  ( 11.25946833292375793, 80.17500000273119554, 8.180482586598731842 ) ) ;
#13595=CARTESIAN_POINT ( 'NONE',  ( 6.987962563135265093, 74.00000000000002842, 12.07036192619727721 ) ) ;
#13600=( BOUNDED_CURVE ( )  B_SPLINE_CURVE ( 2, ( #1892, #27645, #32776, #17353, #19754, #25414, #20272, #25752, #33117, #2236, #4133 ),
 .UNSPECIFIED., .F., .F. ) 
 B_SPLINE_CURVE_WITH_KNOTS ( ( 3, 2, 2, 2, 2, 3 ),
 ( 0.5500000000000000444, 0.5600000000000000533, 0.5799999999999999600, 0.5999999999999999778, 0.6199999999999999956, 0.6250928956683751148 ),
 .UNSPECIFIED. ) 
 CURVE ( )  GEOMETRIC_REPRESENTATION_ITEM ( )  RATIONAL_B_SPLINE_CURVE ( ( 0.9755282581475768211, 0.9755282581475768211, 1.000000000000000000, 0.9510565162951535312, 1.000000000000000000, 0.9510565162951535312, 1.000000000000000000, 0.9510565162951535312, 1.000000000000000000, 0.9875367971922199839, 0.9814209735438224058 ) ) 
 REPRESENTATION_ITEM ( '' )  );
#13607=EDGE_LOOP ( 'NONE', ( #25388, #25278, #24580, #31209 ) ) ;
#13618=CARTESIAN_POINT ( 'NONE',  ( 13.91746824999999532, 79.97500000273115006, -4.522059556121118540 ) ) ;
#13672=CARTESIAN_POINT ( 'NONE',  ( 1.102182119232617911E-15, 102.0000000000000284, 9.000000000000001776 ) ) ;
#13688=CARTESIAN_POINT ( 'NONE',  ( -13.91746824999999532, 78.77500000273117564, -4.522059556121115875 ) ) ;
#13705=ORIENTED_EDGE ( 'NONE', *, *, #27503, .T. ) ;
#13750=CARTESIAN_POINT ( 'NONE',  ( 2.688165632520823219E-15, 79.87500000273114154, 14.63369212191046387 ) ) ;
#13754=CARTESIAN_POINT ( 'NONE',  ( 9.189759918205185230, 74.00000000000001421, 10.46186907115101938 ) ) ;
#13775=VECTOR ( 'NONE', #22675, 1000.000000000000000 ) ;
#13777=CARTESIAN_POINT ( 'NONE',  ( -8.601468415847518756, 78.57500000273120122, -11.83890561707634781 ) ) ;
#13807=ORIENTED_EDGE ( 'NONE', *, *, #33913, .T. ) ;
#13813=CIRCLE ( 'NONE', #15459, 10.64101615137753676 ) ;
#13853=CARTESIAN_POINT ( 'NONE',  ( 9.270509831248425314, 72.95000000546238539, 12.75976212528059683 ) ) ;
#13899=DIRECTION ( 'NONE',  ( -0.000000000000000000, 1.000000000000000000, -0.000000000000000000 ) ) ;
#13901=VECTOR ( 'NONE', #9074, 1000.000000000000000 ) ;
#13905=CARTESIAN_POINT ( 'NONE',  ( -13.91746824999999532, 73.27500000273118985, -4.522059556121115875 ) ) ;
#13918=CARTESIAN_POINT ( 'NONE',  ( -8.960552108402742093E-16, 78.87500000273118417, -14.63369212191046387 ) ) ;
#13923=AXIS2_PLACEMENT_3D ( 'NONE', #13257, #10351, #23224 ) ;
#13944=CARTESIAN_POINT ( 'NONE',  ( 2.688165632520823219E-15, 79.37500000273116996, 14.63369212191046387 ) ) ;
#13983=CARTESIAN_POINT ( 'NONE',  ( 0.000000000000000000, 102.0000000000000284, 14.00000000000000178 ) ) ;
#14016=CARTESIAN_POINT ( 'NONE',  ( 4.300734207923757602, 76.27500000273118985, -13.23629886949340673 ) ) ;
#14022=CARTESIAN_POINT ( 'NONE',  ( -12.13525491562421088, 79.80000000000003979, -8.816778784387096835 ) ) ;
#14024=CIRCLE ( 'NONE', #33183, 15.00000000000000000 ) ;
#14088=CARTESIAN_POINT ( 'NONE',  ( 2.688165632520823219E-15, 73.87500000273116996, 14.63369212191046387 ) ) ;
#14098=CARTESIAN_POINT ( 'NONE',  ( -8.601468415847518756, 81.07500000273117280, -11.83890561707634603 ) ) ;
#14113=CARTESIAN_POINT ( 'NONE',  ( -13.91746824999999532, 78.97500000273117848, 4.522059556121122093 ) ) ;
#14116=EDGE_CURVE ( 'NONE', #26616, #3774, #19717, .T. ) ;
#14141=ORIENTED_EDGE ( 'NONE', *, *, #3157, .F. ) ;
#14183=CARTESIAN_POINT ( 'NONE',  ( 2.688165632520823219E-15, 75.37500000273118417, 14.63369212191046387 ) ) ;
#14189=CARTESIAN_POINT ( 'NONE',  ( -4.223320258572821363E-15, 80.50000000000001421, 15.00000000000000355 ) ) ;
#14252=CARTESIAN_POINT ( 'NONE',  ( -8.601468415847515203, 73.67500000273118133, 11.83890561707634959 ) ) ;
#14262=CARTESIAN_POINT ( 'NONE',  ( 13.91746825000000065, 78.27500000273120406, 4.522059556121115875 ) ) ;
#14270=DIRECTION ( 'NONE',  ( -0.000000000000000000, -1.000000000000000000, -0.000000000000000000 ) ) ;
#14278=CARTESIAN_POINT ( 'NONE',  ( -8.960552108402742093E-16, 78.37500000273119838, -14.63369212191046387 ) ) ;
#14282=ORIENTED_EDGE ( 'NONE', *, *, #21552, .T. ) ;
#14298=ADVANCED_FACE ( 'NONE', ( #15427, #7692 ), #25880, .F. ) ;
#14350=CARTESIAN_POINT ( 'NONE',  ( -8.601468415847515203, 75.17500000273118133, 11.83890561707634959 ) ) ;
#14356=CARTESIAN_POINT ( 'NONE',  ( -23.09401076758502924, 96.00000000000002842, 5.354274672883389237E-15 ) ) ;
#14378=CARTESIAN_POINT ( 'NONE',  ( -8.749005742281003251, 74.00000000000004263, 11.56706244653782001 ) ) ;
#14384=SURFACE_STYLE_USAGE ( .BOTH. , #26756 ) ;
#14410=AXIS2_PLACEMENT_3D ( 'NONE', #33574, #15745, #12299 ) ;
#14422=CARTESIAN_POINT ( 'NONE',  ( -12.13525491562420910, 80.19999999999998863, 8.816778784387098611 ) ) ;
#14431=CARTESIAN_POINT ( 'NONE',  ( 11.25946833292375793, 80.57500000273121543, -8.180482586598735395 ) ) ;
#14433=CARTESIAN_POINT ( 'NONE',  ( -9.657523855033125146E-16, 79.75000000546238255, -15.77193336357400710 ) ) ;
#14437=CARTESIAN_POINT ( 'NONE',  ( 0.000000000000000000, 74.00000000000001421, 0.000000000000000000 ) ) ;
#14445=CARTESIAN_POINT ( 'NONE',  ( 11.25946833292375793, 72.07500000273120122, -8.180482586598735395 ) ) ;
#14455=VECTOR ( 'NONE', #16565, 1000.000000000000114 ) ;
#14461=APPLICATION_CONTEXT ( 'automotive_design' ) ;
#14506=CARTESIAN_POINT ( 'NONE',  ( 0.000000000000000000, 74.00000000000001421, 0.000000000000000000 ) ) ;
#14517=CARTESIAN_POINT ( 'NONE',  ( 4.300734207923761154, 75.47500000273116427, 13.23629886949340495 ) ) ;
#14527=CARTESIAN_POINT ( 'NONE',  ( -2.375766604868048137, 78.44874571845311095, 14.99999999999999822 ) ) ;
#14533=ORIENTED_EDGE ( 'NONE', *, *, #33247, .T. ) ;
#14549=DIRECTION ( 'NONE',  ( -0.4999999999999997224, 0.000000000000000000, 0.8660254037844388186 ) ) ;
#14590=CARTESIAN_POINT ( 'NONE',  ( 4.635254915624212657, 80.60000000000000853, 14.26584774442730286 ) ) ;
#14601=CARTESIAN_POINT ( 'NONE',  ( -8.601468415847518756, 77.07500000273118701, -11.83890561707634603 ) ) ;
#14603=CARTESIAN_POINT ( 'NONE',  ( 12.13525491562421088, 79.05000000546236549, 8.816778784387095058 ) ) ;
#14616=CARTESIAN_POINT ( 'NONE',  ( -11.25946833292375793, 81.17500000273119554, -8.180482586598733619 ) ) ;
#14671=CARTESIAN_POINT ( 'NONE',  ( -15.00000000000000000, 76.09999999999998010, 4.873795443493597723 ) ) ;
#14689=CARTESIAN_POINT ( 'NONE',  ( 4.300734207923757602, 72.27500000273117564, -13.23629886949340673 ) ) ;
#14699=CARTESIAN_POINT ( 'NONE',  ( -12.13525491562420910, 78.19999999999998863, 8.816778784387098611 ) ) ;
#14708=EDGE_LOOP ( 'NONE', ( #14141, #17323, #31797, #12686 ) ) ;
#14732=CARTESIAN_POINT ( 'NONE',  ( 11.54700538379251817, 96.00000000000002842, 19.99999999999999645 ) ) ;
#14758=CARTESIAN_POINT ( 'NONE',  ( -13.91746824999999887, 75.37500000273116996, 0.000000000000000000 ) ) ;
#14770=CARTESIAN_POINT ( 'NONE',  ( 15.00000000000000000, 75.25000000546239676, -1.836970198721029589E-15 ) ) ;
#14782=CARTESIAN_POINT ( 'NONE',  ( 11.25946833292375793, 80.17500000273119554, 8.180482586598731842 ) ) ;
#14823=ADVANCED_FACE ( 'NONE', ( #29538 ), #24317, .T. ) ;
#14857=CARTESIAN_POINT ( 'NONE',  ( -8.891200544363830713E-16, 75.50000000000001421, -15.00000000000000000 ) ) ;
#14866=CARTESIAN_POINT ( 'NONE',  ( -4.635254915624211769, 77.60000000000000853, -14.26584774442730286 ) ) ;
#14876=ADVANCED_FACE ( 'NONE', ( #13578 ), #24371, .T. ) ;
#14882=FACE_OUTER_BOUND ( 'NONE', #13607, .T. ) ;
#14930=CARTESIAN_POINT ( 'NONE',  ( -9.270509831248425314, 73.70000000000000284, -12.75976212528059861 ) ) ;
#14942=CARTESIAN_POINT ( 'NONE',  ( 15.00000000000000000, 79.35000000546241949, -4.873795443493596835 ) ) ;
#14954=CARTESIAN_POINT ( 'NONE',  ( -8.960552108402744065E-16, 80.37500000273119838, -14.63369212191046209 ) ) ;
#14957=CARTESIAN_POINT ( 'NONE',  ( -4.300734207923759378, 74.47500000273116427, -13.23629886949340495 ) ) ;
#14961=CARTESIAN_POINT ( 'NONE',  ( 12.13525491562421088, 78.80000000000003979, 8.816778784387095058 ) ) ;
#14984=ORIENTED_EDGE ( 'NONE', *, *, #29583, .F. ) ;
#15000=AXIS2_PLACEMENT_3D ( 'NONE', #33447, #21302, #15812 ) ;
#15010=LINE ( 'NONE', #9166, #11566 ) ;
#15027=ADVANCED_FACE ( 'NONE', ( #8347 ), #15589, .T. ) ;
#15033=CARTESIAN_POINT ( 'NONE',  ( 11.25946833292375793, 71.67500000273119554, 8.180482586598731842 ) ) ;
#15052=EDGE_LOOP ( 'NONE', ( #28890, #14533, #21100, #24724 ) ) ;
#15062=CARTESIAN_POINT ( 'NONE',  ( -1.877258788446258597, 74.00000000000004263, 14.08662250695439155 ) ) ;
#15105=CARTESIAN_POINT ( 'NONE',  ( 15.00000000000000000, 77.10000000000000853, -4.873795443493596835 ) ) ;
#15117=CARTESIAN_POINT ( 'NONE',  ( 9.270509831248425314, 74.95000000546237118, 12.75976212528059683 ) ) ;
#15132=CARTESIAN_POINT ( 'NONE',  ( -13.91746824999999887, 70.87500000273122680, 0.000000000000000000 ) ) ;
#15137=CARTESIAN_POINT ( 'NONE',  ( -1.089172066684569321E-14, 78.49999999999998579, 15.00000000000000000 ) ) ;
#15140=ORIENTED_EDGE ( 'NONE', *, *, #12795, .F. ) ;
#15177=CARTESIAN_POINT ( 'NONE',  ( 0.000000000000000000, 111.9999999999999858, 0.000000000000000000 ) ) ;
#15197=CARTESIAN_POINT ( 'NONE',  ( 2.375766604868043697, 80.55125428154687484, 15.00000000000000178 ) ) ;
#15204=CARTESIAN_POINT ( 'NONE',  ( 4.635254915624209993, 75.40000000000001990, -14.26584774442730463 ) ) ;
#15262=VERTEX_POINT ( 'NONE', #23982 ) ;
#15275=CARTESIAN_POINT ( 'NONE',  ( 4.635254915624212657, 74.59999999999999432, 14.26584774442730286 ) ) ;
#15285=CARTESIAN_POINT ( 'NONE',  ( -8.601468415847518756, 75.07500000273118701, -11.83890561707634603 ) ) ;
#15287=CARTESIAN_POINT ( 'NONE',  ( -8.960552108402742093E-16, 80.37500000273118417, -14.63369212191046387 ) ) ;
#15300=CARTESIAN_POINT ( 'NONE',  ( -8.601468415847518756, 79.07500000273118701, -11.83890561707634781 ) ) ;
#15309=ORIENTED_EDGE ( 'NONE', *, *, #1942, .T. ) ;
#15371=CARTESIAN_POINT ( 'NONE',  ( 8.891200544363830713E-16, 81.50000000000001421, -15.00000000000000000 ) ) ;
#15378=PRODUCT_DEFINITION_SHAPE ( 'NONE', 'NONE',  #18358 ) ;
#15379=CARTESIAN_POINT ( 'NONE',  ( 4.635254915624212657, 74.59999999999999432, 14.26584774442730286 ) ) ;
#15398=CYLINDRICAL_SURFACE ( 'NONE', #23757, 12.00000000000000178 ) ;
#15427=FACE_BOUND ( 'NONE', #30055, .T. ) ;
#15448=CARTESIAN_POINT ( 'NONE',  ( 4.635254915624212657, 76.59999999999999432, 14.26584774442730286 ) ) ;
#15459=AXIS2_PLACEMENT_3D ( 'NONE', #19823, #33013, #27212 ) ;
#15472=CARTESIAN_POINT ( 'NONE',  ( -8.960552108402744065E-16, 74.37500000273121259, -14.63369212191046209 ) ) ;
#15475=CARTESIAN_POINT ( 'NONE',  ( -13.91746824999999532, 75.27500000273118985, -4.522059556121115875 ) ) ;
#15476=PRESENTATION_STYLE_ASSIGNMENT (( #19639 ) ) ;
#15506=( BOUNDED_CURVE ( )  B_SPLINE_CURVE ( 2, ( #4364, #25127, #16908, #22387, #24955, #32836, #17245 ),
 .UNSPECIFIED., .F., .T. ) 
 B_SPLINE_CURVE_WITH_KNOTS ( ( 3, 2, 2, 3 ),
 ( 0.7500000000000000000, 0.7600000000000001199, 0.7800000000000004707, 0.8000000000000007105 ),
 .UNSPECIFIED. ) 
 CURVE ( )  GEOMETRIC_REPRESENTATION_ITEM ( )  RATIONAL_B_SPLINE_CURVE ( ( 0.9755282581475768211, 0.9755282581475768211, 1.000000000000000000, 0.9510565162951535312, 1.000000000000000000, 0.9510565162951518658, 1.000000000000001554 ) ) 
 REPRESENTATION_ITEM ( '' )  );
#15531=EDGE_LOOP ( 'NONE', ( #9126, #25896 ) ) ;
#15533=CIRCLE ( 'NONE', #33028, 9.000000000000001776 ) ;
#15560=FACE_OUTER_BOUND ( 'NONE', #27327, .T. ) ;
#15589=CYLINDRICAL_SURFACE ( 'NONE', #5097, 15.00000000000000000 ) ;
#15597=DIRECTION ( 'NONE',  ( -0.000000000000000000, 1.000000000000000000, -0.000000000000000000 ) ) ;
#15609=EDGE_CURVE ( 'NONE', #23625, #22018, #12433, .T. ) ;
#15626=CARTESIAN_POINT ( 'NONE',  ( 9.270509831248425314, 78.70000000000003126, 12.75976212528059683 ) ) ;
#15636=CARTESIAN_POINT ( 'NONE',  ( 12.41655794490159082, 74.00000000000001421, -6.419367199009562874 ) ) ;
#15638=FACE_OUTER_BOUND ( 'NONE', #18058, .T. ) ;
#15646=CARTESIAN_POINT ( 'NONE',  ( 13.91746824999999532, 75.97500000273116427, -4.522059556121118540 ) ) ;
#15650=CARTESIAN_POINT ( 'NONE',  ( -4.300734207923759378, 74.97500000273122112, -13.23629886949340495 ) ) ;
#15696=LINE ( 'NONE', #26150, #27631 ) ;
#15745=DIRECTION ( 'NONE',  ( 0.000000000000000000, 1.000000000000000000, 0.000000000000000000 ) ) ;
#15751=ADVANCED_FACE ( 'NONE', ( #1792, #30109 ), #25493, .T. ) ;
#15787=ORIENTED_EDGE ( 'NONE', *, *, #29234, .T. ) ;
#15793=CARTESIAN_POINT ( 'NONE',  ( 4.635254915624209993, 73.40000000000001990, -14.26584774442730463 ) ) ;
#15802=CARTESIAN_POINT ( 'NONE',  ( 9.081462083391590667, 73.99999999999997158, -10.89876187695312915 ) ) ;
#15812=DIRECTION ( 'NONE',  ( -0.4999999999999996669, 0.000000000000000000, 0.8660254037844388186 ) ) ;
#15813=CARTESIAN_POINT ( 'NONE',  ( -13.91746824999999532, 76.97500000273119269, 4.522059556121122093 ) ) ;
#15816=CIRCLE ( 'NONE', #16350, 14.00000000000000178 ) ;
#15817=CARTESIAN_POINT ( 'NONE',  ( -8.601468415847518756, 77.07500000273117280, -11.83890561707634781 ) ) ;
#15863=ORIENTED_EDGE ( 'NONE', *, *, #22368, .F. ) ;
#15897=ADVANCED_FACE ( 'NONE', ( #21833 ), #11683, .T. ) ;
#15914=DIRECTION ( 'NONE',  ( -0.000000000000000000, -1.000000000000000000, -0.000000000000000000 ) ) ;
#15933=CARTESIAN_POINT ( 'NONE',  ( -13.91746824999999887, 78.87500000273118417, 0.000000000000000000 ) ) ;
#15946=EDGE_CURVE ( 'NONE', #29890, #9461, #4760, .T. ) ;
#15960=CARTESIAN_POINT ( 'NONE',  ( 9.270509831248423538, 73.30000000000001137, -12.75976212528059861 ) ) ;
#15978=AXIS2_PLACEMENT_3D ( 'NONE', #11142, #3743, #21781 ) ;
#15982=CARTESIAN_POINT ( 'NONE',  ( -11.25946833292375793, 79.07500000273121543, 8.180482586598737171 ) ) ;
#15986=CARTESIAN_POINT ( 'NONE',  ( 11.25946833292375793, 76.17500000273119554, 8.180482586598731842 ) ) ;
#15988=EDGE_CURVE ( 'NONE', #30053, #17164, #21995, .T. ) ;
#16000=CARTESIAN_POINT ( 'NONE',  ( 8.601468415847516980, 76.67500000273118133, -11.83890561707634781 ) ) ;
#16002=CARTESIAN_POINT ( 'NONE',  ( -15.00000000000000000, 76.25000000546239676, 0.000000000000000000 ) ) ;
#16005=CARTESIAN_POINT ( 'NONE',  ( 0.000000000000000000, 102.0000000000000284, 0.000000000000000000 ) ) ;
#16019=DIRECTION ( 'NONE',  ( 0.000000000000000000, 1.000000000000000000, 0.000000000000000000 ) ) ;
#16035=CARTESIAN_POINT ( 'NONE',  ( 15.00000000000000000, 77.10000000000000853, -4.873795443493596835 ) ) ;
#16038=ORIENTED_EDGE ( 'NONE', *, *, #9244, .T. ) ;
#16106=CARTESIAN_POINT ( 'NONE',  ( -4.300734207923755825, 79.27500000273118985, 13.23629886949340673 ) ) ;
#16153=CARTESIAN_POINT ( 'NONE',  ( 4.300734207923761154, 75.47500000273116427, 13.23629886949340495 ) ) ;
#16169=CARTESIAN_POINT ( 'NONE',  ( 4.300734207923761154, 75.97500000273122112, 13.23629886949340495 ) ) ;
#16171=CARTESIAN_POINT ( 'NONE',  ( -9.270509831248423538, 75.95000000546239960, -12.75976212528059861 ) ) ;
#16187=DIRECTION ( 'NONE',  ( 0.000000000000000000, 0.000000000000000000, 1.000000000000000000 ) ) ;
#16211=ORIENTED_EDGE ( 'NONE', *, *, #29912, .T. ) ;
#16213=CARTESIAN_POINT ( 'NONE',  ( -14.45873412499999944, 80.56250000409676204, 0.000000000000000000 ) ) ;
#16249=ORIENTED_EDGE ( 'NONE', *, *, #23732, .T. ) ;
#16268=CARTESIAN_POINT ( 'NONE',  ( 11.25946833292375793, 80.07500000273121543, -8.180482586598735395 ) ) ;
#16291=LINE ( 'NONE', #647, #23426 ) ;
#16303=EDGE_CURVE ( 'NONE', #16782, #26616, #24399, .T. ) ;
#16306=CARTESIAN_POINT ( 'NONE',  ( 11.56287504972942592, 74.00000000000000000, -7.975283324587876699 ) ) ;
#16315=DIRECTION ( 'NONE',  ( 0.000000000000000000, 0.000000000000000000, 1.000000000000000000 ) ) ;
#16334=CARTESIAN_POINT ( 'NONE',  ( -13.91746824999999532, 81.27500000273117564, -4.522059556121115875 ) ) ;
#16338=CARTESIAN_POINT ( 'NONE',  ( 13.44965385310867312, 74.00000000000005684, 3.606845949684043706 ) ) ;
#16348=EDGE_LOOP ( 'NONE', ( #21605, #17280 ) ) ;
#16350=AXIS2_PLACEMENT_3D ( 'NONE', #27224, #3225, #29786 ) ;
#16375=VERTEX_POINT ( 'NONE', #17187 ) ;
#16412=EDGE_CURVE ( 'NONE', #19608, #17758, #13600, .T. ) ;
#16434=CARTESIAN_POINT ( 'NONE',  ( 4.300734207923761154, 79.47500000273116427, 13.23629886949340495 ) ) ;
#16439=CARTESIAN_POINT ( 'NONE',  ( -9.270509831248423538, 79.95000000546238539, -12.75976212528059861 ) ) ;
#16443=FACE_OUTER_BOUND ( 'NONE', #6937, .T. ) ;
#16451=ORIENTED_EDGE ( 'NONE', *, *, #21264, .T. ) ;
#16454=CARTESIAN_POINT ( 'NONE',  ( 1.836970198721029589E-15, 74.00000000000001421, -15.00000000000000000 ) ) ;
#16481=ORIENTED_EDGE ( 'NONE', *, *, #28656, .F. ) ;
#16494=CARTESIAN_POINT ( 'NONE',  ( 4.300734207923761154, 79.97500000273122112, 13.23629886949340495 ) ) ;
#16521=CARTESIAN_POINT ( 'NONE',  ( 4.300734207923757602, 80.27500000273118985, -13.23629886949340673 ) ) ;
#16536=EDGE_LOOP ( 'NONE', ( #29868, #7784, #6223, #5562 ) ) ;
#16565=DIRECTION ( 'NONE',  ( -0.5000000000000002220, 0.000000000000000000, -0.8660254037844384856 ) ) ;
#16586=CARTESIAN_POINT ( 'NONE',  ( 15.00000000000000000, 77.35000000546233423, -4.873795443493596835 ) ) ;
#16596=CARTESIAN_POINT ( 'NONE',  ( 8.601468415847516980, 78.17500000273120975, -11.83890561707634781 ) ) ;
#16664=CARTESIAN_POINT ( 'NONE',  ( 8.601468415847516980, 80.67500000273118133, -11.83890561707634781 ) ) ;
#16672=LINE ( 'NONE', #32769, #11809 ) ;
#16673=CARTESIAN_POINT ( 'NONE',  ( 8.601468415847516980, 76.67500000273118133, -11.83890561707634603 ) ) ;
#16688=CARTESIAN_POINT ( 'NONE',  ( 8.601468415847516980, 80.17500000273113869, -11.83890561707634781 ) ) ;
#16747=CARTESIAN_POINT ( 'NONE',  ( 4.635254915624209993, 75.65000000546234560, -14.26584774442730463 ) ) ;
#16761=CARTESIAN_POINT ( 'NONE',  ( -11.25946833292375793, 73.07500000273120122, 8.180482586598737171 ) ) ;
#16782=VERTEX_POINT ( 'NONE', #21792 ) ;
#16798=SHAPE_REPRESENTATION_RELATIONSHIP ( 'NONE' , 'NONE' ,  #3268, #29162 ) ;
#16803=( BOUNDED_CURVE ( )  B_SPLINE_CURVE ( 2, ( #32344, #3696, #16747, #19488, #18993, #777, #5938, #6441, #24626, #11419, #29437, #1099, #8838 ),
 .UNSPECIFIED., .F., .T. ) 
 B_SPLINE_CURVE_WITH_KNOTS ( ( 3, 2, 2, 2, 2, 2, 3 ),
 ( 0.4500000000000000111, 0.4600000000000000200, 0.4799999999999999822, 0.5000000000000000000, 0.5200000000000000178, 0.5400000000000000355, 0.5500000000000000444 ),
 .UNSPECIFIED. ) 
 CURVE ( )  GEOMETRIC_REPRESENTATION_ITEM ( )  RATIONAL_B_SPLINE_CURVE ( ( 0.9755282581475768211, 0.9755282581475768211, 1.000000000000000000, 0.9510565162951535312, 1.000000000000000000, 0.9510565162951535312, 1.000000000000000000, 0.9510565162951535312, 1.000000000000000000, 0.9510565162951535312, 1.000000000000000000, 0.9755282581475768211, 0.9755282581475768211 ) ) 
 REPRESENTATION_ITEM ( '' )  );
#16819=CARTESIAN_POINT ( 'NONE',  ( 1.469576158976824144E-15, 102.0000000000000284, 12.00000000000000178 ) ) ;
#16834=CARTESIAN_POINT ( 'NONE',  ( 11.25946833292375793, 72.57500000273120122, -8.180482586598735395 ) ) ;
#16843=CARTESIAN_POINT ( 'NONE',  ( -13.91746824999999532, 81.27500000273117564, -4.522059556121115875 ) ) ;
#16847=ORIENTED_EDGE ( 'NONE', *, *, #16412, .T. ) ;
#16866=EDGE_LOOP ( 'NONE', ( #12595, #11579, #26825, #24299, #11256, #13503 ) ) ;
#16894=CARTESIAN_POINT ( 'NONE',  ( -2.375766604868044141, 81.55125428154683220, -14.99999999999999822 ) ) ;
#16908=CARTESIAN_POINT ( 'NONE',  ( -4.635254915624208216, 74.40000000000001990, 14.26584774442730463 ) ) ;
#16930=CARTESIAN_POINT ( 'NONE',  ( -8.601468415847515203, 77.17500000273118133, 11.83890561707634959 ) ) ;
#16977=CARTESIAN_POINT ( 'NONE',  ( 0.000000000000000000, 74.00000000000001421, 0.000000000000000000 ) ) ;
#16999=CARTESIAN_POINT ( 'NONE',  ( 13.91746824999999887, 74.37500000273116996, -1.704398294459741270E-15 ) ) ;
#17009=CARTESIAN_POINT ( 'NONE',  ( -13.91746824999999532, 77.47500000273117848, 4.522059556121122093 ) ) ;
#17024=CARTESIAN_POINT ( 'NONE',  ( -8.960552108402742093E-16, 76.37500000273114154, -14.63369212191046387 ) ) ;
#17034=EDGE_LOOP ( 'NONE', ( #31836, #8630, #25037, #7140 ) ) ;
#17044=LINE ( 'NONE', #27340, #4707 ) ;
#17080=CARTESIAN_POINT ( 'NONE',  ( -8.891200544363830713E-16, 75.50000000000001421, -15.00000000000000000 ) ) ;
#17097=CARTESIAN_POINT ( 'NONE',  ( -11.25946833292375793, 76.67500000273119554, -8.180482586598733619 ) ) ;
#17129=CARTESIAN_POINT ( 'NONE',  ( -11.79757697019589457, 74.00000000000001421, 8.763667255710268833 ) ) ;
#17163=CARTESIAN_POINT ( 'NONE',  ( 0.000000000000000000, 74.00000000000001421, 15.00000000000000000 ) ) ;
#17164=VERTEX_POINT ( 'NONE', #24159 ) ;
#17167=VECTOR ( 'NONE', #15597, 1000.000000000000000 ) ;
#17171=CARTESIAN_POINT ( 'NONE',  ( 8.601468415847520532, 72.07500000273117280, 11.83890561707634781 ) ) ;
#17179=CARTESIAN_POINT ( 'NONE',  ( 0.000000000000000000, 74.00000000000001421, 0.000000000000000000 ) ) ;
#17180=CARTESIAN_POINT ( 'NONE',  ( -4.300734207923759378, 76.97500000273122112, -13.23629886949340495 ) ) ;
#17182=CARTESIAN_POINT ( 'NONE',  ( 4.635254915624209993, 75.65000000546234560, -14.26584774442730463 ) ) ;
#17187=CARTESIAN_POINT ( 'NONE',  ( 12.86449124955741041, 74.00000000000001421, -5.310441354522136947 ) ) ;
#17195=CARTESIAN_POINT ( 'NONE',  ( -13.91746824999999887, 72.87500000273122680, 0.000000000000000000 ) ) ;
#17199=CARTESIAN_POINT ( 'NONE',  ( 9.270509831248421762, 79.29999999999999716, -12.75976212528059861 ) ) ;
#17205=EDGE_CURVE ( 'NONE', #11228, #19151, #23994, .T. ) ;
#17210=EDGE_CURVE ( 'NONE', #8282, #22733, #29803, .T. ) ;
#17215=CARTESIAN_POINT ( 'NONE',  ( 12.13525491562420910, 77.45000000546237118, -8.816778784387098611 ) ) ;
#17245=CARTESIAN_POINT ( 'NONE',  ( -15.00000000000000000, 74.00000000000001421, 0.000000000000000000 ) ) ;
#17264=CARTESIAN_POINT ( 'NONE',  ( -11.25946833292375793, 75.07500000273120122, 8.180482586598737171 ) ) ;
#17274=CARTESIAN_POINT ( 'NONE',  ( -15.00000000000000000, 77.89999999999997726, -4.873795443493594171 ) ) ;
#17280=ORIENTED_EDGE ( 'NONE', *, *, #31175, .T. ) ;
#17323=ORIENTED_EDGE ( 'NONE', *, *, #19726, .F. ) ;
#17337=CARTESIAN_POINT ( 'NONE',  ( -11.25946833292375793, 75.57500000273120122, 8.180482586598737171 ) ) ;
#17346=CARTESIAN_POINT ( 'NONE',  ( 4.300734207923761154, 75.97500000273122112, 13.23629886949340495 ) ) ;
#17348=CARTESIAN_POINT ( 'NONE',  ( -15.00000000000000000, 78.15000000546238823, -4.873795443493594171 ) ) ;
#17353=CARTESIAN_POINT ( 'NONE',  ( -9.270509831248419985, 74.55000000546237970, 12.75976212528060039 ) ) ;
#17361=CARTESIAN_POINT ( 'NONE',  ( -4.300734207923755825, 75.27500000273118985, 13.23629886949340673 ) ) ;
#17395=DIRECTION ( 'NONE',  ( -0.8660254037844385966, 0.000000000000000000, 0.5000000000000003331 ) ) ;
#17411=VERTEX_POINT ( 'NONE', #28072 ) ;
#17422=FACE_OUTER_BOUND ( 'NONE', #9105, .T. ) ;
#17456=ORIENTED_EDGE ( 'NONE', *, *, #33247, .F. ) ;
#17469=CARTESIAN_POINT ( 'NONE',  ( -14.73595198987283972, 73.99999999999997158, 2.369153449599709305 ) ) ;
#17496=VERTEX_POINT ( 'NONE', #14356 ) ;
#17509=CARTESIAN_POINT ( 'NONE',  ( -15.00000000000000000, 73.90000000000000568, -4.873795443493594171 ) ) ;
#17518=CARTESIAN_POINT ( 'NONE',  ( 8.959971004064378519, 74.08848768517671601, 11.34546913621253950 ) ) ;
#17520=CARTESIAN_POINT ( 'NONE',  ( 15.00000000000000000, 77.25000000546239676, -1.836970198721029589E-15 ) ) ;
#17530=CARTESIAN_POINT ( 'NONE',  ( -4.300734207923759378, 80.47500000273116427, -13.23629886949340495 ) ) ;
#17533=CARTESIAN_POINT ( 'NONE',  ( 11.25946833292375793, 74.07500000273120122, -8.180482586598735395 ) ) ;
#17538=CARTESIAN_POINT ( 'NONE',  ( -23.09401076758502924, 96.00000000000002842, 5.354274672883389237E-15 ) ) ;
#17544=ORIENTED_EDGE ( 'NONE', *, *, #30831, .F. ) ;
#17545=EDGE_CURVE ( 'NONE', #28806, #8605, #30121, .T. ) ;
#17581=EDGE_LOOP ( 'NONE', ( #29584, #3237, #20412, #3134, #20460, #26961, #20327, #29409 ) ) ;
#17614=CARTESIAN_POINT ( 'NONE',  ( -1.089172066684569321E-14, 78.49999999999998579, 15.00000000000000000 ) ) ;
#17636=PLANE ( 'NONE',  #27490 ) ;
#17637=CARTESIAN_POINT ( 'NONE',  ( -14.28731510817884498, 73.99999999999998579, 4.080734695941037771 ) ) ;
#17642=ADVANCED_FACE ( 'NONE', ( #15560 ), #26013, .F. ) ;
#17656=DIRECTION ( 'NONE',  ( 0.000000000000000000, -0.000000000000000000, 1.000000000000000000 ) ) ;
#17672=CIRCLE ( 'NONE', #9442, 13.32050807568876927 ) ;
#17678=CARTESIAN_POINT ( 'NONE',  ( 4.635254915624209993, 77.39999999999996305, -14.26584774442730463 ) ) ;
#17692=CARTESIAN_POINT ( 'NONE',  ( -12.13525491562420910, 76.45000000546237118, 8.816778784387098611 ) ) ;
#17697=AXIS2_PLACEMENT_3D ( 'NONE', #16977, #119, #10275 ) ;
#17706=CARTESIAN_POINT ( 'NONE',  ( 13.91746825000000065, 73.77500000273116143, 4.522059556121114987 ) ) ;
#17758=VERTEX_POINT ( 'NONE', #12803 ) ;
#17773=CARTESIAN_POINT ( 'NONE',  ( 15.00000000000000355, 80.90000000000000568, 4.873795443493592394 ) ) ;
#17780=CARTESIAN_POINT ( 'NONE',  ( 15.00000000000000000, 75.00000000000001421, -1.836970198721029589E-15 ) ) ;
#17791=MECHANICAL_DESIGN_GEOMETRIC_PRESENTATION_REPRESENTATION('',(#31478),#29820);
#17802=CARTESIAN_POINT ( 'NONE',  ( 0.000000000000000000, 102.0000000000000284, 14.00000000000000178 ) ) ;
#17814=CARTESIAN_POINT ( 'NONE',  ( -1.550433958383848148E-15, 111.9999999999999858, -11.32050807568876749 ) ) ;
#17827=CARTESIAN_POINT ( 'NONE',  ( 0.000000000000000000, 102.0000000000000284, 0.000000000000000000 ) ) ;
#17856=CARTESIAN_POINT ( 'NONE',  ( 4.635254915624209993, 75.40000000000001990, -14.26584774442730463 ) ) ;
#17868=CARTESIAN_POINT ( 'NONE',  ( -4.635254915624208216, 76.65000000546234560, 14.26584774442730463 ) ) ;
#17882=CARTESIAN_POINT ( 'NONE',  ( 13.91746824999999887, 73.87500000273116996, -1.704398294459741270E-15 ) ) ;
#17888=CARTESIAN_POINT ( 'NONE',  ( 2.375766604868040144, 78.55125428154684641, 15.00000000000000178 ) ) ;
#17935=DIRECTION ( 'NONE',  ( 0.000000000000000000, 0.000000000000000000, 1.000000000000000000 ) ) ;
#17978=DIRECTION ( 'NONE',  ( 0.000000000000000000, 0.000000000000000000, -1.000000000000000000 ) ) ;
#17994=EDGE_CURVE ( 'NONE', #9084, #29760, #19140, .T. ) ;
#18017=EDGE_LOOP ( 'NONE', ( #21394, #8748, #8160, #32290 ) ) ;
#18029=CARTESIAN_POINT ( 'NONE',  ( 15.00000000000000355, 76.90000000000000568, 4.873795443493592394 ) ) ;
#18040=CARTESIAN_POINT ( 'NONE',  ( -13.91746824999999532, 75.47500000273116427, 4.522059556121122093 ) ) ;
#18052=CARTESIAN_POINT ( 'NONE',  ( -8.601468415847515203, 73.67500000273118133, 11.83890561707634959 ) ) ;
#18058=EDGE_LOOP ( 'NONE', ( #2390, #24823, #6197, #22548 ) ) ;
#18066=CARTESIAN_POINT ( 'NONE',  ( -12.13525491562420910, 76.45000000546237118, 8.816778784387098611 ) ) ;
#18079=EDGE_CURVE ( 'NONE', #22980, #22878, #24445, .T. ) ;
#18121=EDGE_CURVE ( 'NONE', #10457, #25891, #33750, .T. ) ;
#18173=CARTESIAN_POINT ( 'NONE',  ( -13.91746824999999887, 81.12500000273121259, 0.000000000000000000 ) ) ;
#18177=CARTESIAN_POINT ( 'NONE',  ( 0.000000000000000000, 86.00000000000001421, 0.000000000000000000 ) ) ;
#18191=EDGE_LOOP ( 'NONE', ( #8123, #13705, #22860, #14984, #24168, #2808, #25582, #15863, #17544, #33715 ) ) ;
#18199=CARTESIAN_POINT ( 'NONE',  ( 12.13525491562420910, 75.19999999999998863, -8.816778784387098611 ) ) ;
#18222=CARTESIAN_POINT ( 'NONE',  ( -8.601468415847518756, 78.57500000273120122, -11.83890561707634603 ) ) ;
#18225=CARTESIAN_POINT ( 'NONE',  ( 4.300734207923761154, 79.97500000273122112, 13.23629886949340495 ) ) ;
#18278=VERTEX_POINT ( 'NONE', #23018 ) ;
#18292=CARTESIAN_POINT ( 'NONE',  ( 15.00000000000000000, 81.00000000000001421, -1.836970198721029589E-15 ) ) ;
#18358=PRODUCT_DEFINITION ( 'UNKNOWN', '', #9324, #31903 ) ;
#18367=STYLED_ITEM ( 'NONE', ( #15476 ), #32070 ) ;
#18378=CARTESIAN_POINT ( 'NONE',  ( 2.013924091267699445, 74.00000000000002842, -14.36055101182497040 ) ) ;
#18388=CARTESIAN_POINT ( 'NONE',  ( -13.91746824999999532, 78.97500000273117848, 4.522059556121122093 ) ) ;
#18391=CARTESIAN_POINT ( 'NONE',  ( -13.91746824999999887, 79.37500000273118417, 0.000000000000000000 ) ) ;
#18426=ORIENTED_EDGE ( 'NONE', *, *, #30738, .F. ) ;
#18507=EDGE_CURVE ( 'NONE', #26616, #5592, #19503, .T. ) ;
#18510=CARTESIAN_POINT ( 'NONE',  ( -13.91746824999999532, 80.77500000273118985, -4.522059556121115875 ) ) ;
#18514=EDGE_CURVE ( 'NONE', #15262, #16375, #20205, .T. ) ;
#18533=DIRECTION ( 'NONE',  ( -1.000000000000000000, 0.000000000000000000, -0.000000000000000000 ) ) ;
#18537=CARTESIAN_POINT ( 'NONE',  ( -4.635254915624211769, 73.59999999999999432, -14.26584774442730286 ) ) ;
#18546=CARTESIAN_POINT ( 'NONE',  ( 4.841599045666881374, 74.00000000000004263, -13.55140770215843027 ) ) ;
#18557=CARTESIAN_POINT ( 'NONE',  ( 13.91746825000000065, 79.77500000273116143, 4.522059556121115875 ) ) ;
#18561=CARTESIAN_POINT ( 'NONE',  ( 8.601468415847516980, 78.67500000273119554, -11.83890561707634781 ) ) ;
#18578=CARTESIAN_POINT ( 'NONE',  ( -8.601468415847518756, 79.07500000273118701, -11.83890561707634781 ) ) ;
#18582=CARTESIAN_POINT ( 'NONE',  ( 10.49071758506610763, 74.00000000000000000, 9.190572033506278160 ) ) ;
#18673=CARTESIAN_POINT ( 'NONE',  ( 0.000000000000000000, 74.00000000000001421, 0.000000000000000000 ) ) ;
#18679=CARTESIAN_POINT ( 'NONE',  ( -9.657523855033125146E-16, 73.75000000546233991, -15.77193336357400710 ) ) ;
#18681=CARTESIAN_POINT ( 'NONE',  ( 2.688165632520823219E-15, 77.87500000273119838, 14.63369212191046387 ) ) ;
#18703=VERTEX_POINT ( 'NONE', #33258 ) ;
#18728=CARTESIAN_POINT ( 'NONE',  ( 11.25946833292375793, 77.67500000273119554, 8.180482586598731842 ) ) ;
#18731=CARTESIAN_POINT ( 'NONE',  ( -4.300734207923759378, 72.97500000273122112, -13.23629886949340495 ) ) ;
#18744=CARTESIAN_POINT ( 'NONE',  ( 11.25946833292375793, 78.57500000273121543, -8.180482586598735395 ) ) ;
#18748=FACE_OUTER_BOUND ( 'NONE', #22593, .T. ) ;
#18759=ORIENTED_EDGE ( 'NONE', *, *, #26240, .T. ) ;
#18782=ORIENTED_EDGE ( 'NONE', *, *, #26576, .T. ) ;
#18841=CARTESIAN_POINT ( 'NONE',  ( -11.25946833292375793, 80.67500000273119554, -8.180482586598733619 ) ) ;
#18846=CARTESIAN_POINT ( 'NONE',  ( 8.891200544363830713E-16, 79.75000000546238255, -15.00000000000000000 ) ) ;
#18847=CARTESIAN_POINT ( 'NONE',  ( -15.00000000000000000, 79.89999999999997726, -4.873795443493594171 ) ) ;
#18876=CARTESIAN_POINT ( 'NONE',  ( 0.2410918355672596325, 74.00000000000002842, -14.56788933630795491 ) ) ;
#18885=UNCERTAINTY_MEASURE_WITH_UNIT (LENGTH_MEASURE( 1.000000000000000082E-05 ), #6321, 'distance_accuracy_value', 'NONE');
#18890=CARTESIAN_POINT ( 'NONE',  ( -8.601468415847518756, 74.57500000273120122, -11.83890561707634603 ) ) ;
#18893=CARTESIAN_POINT ( 'NONE',  ( 8.601468415847520532, 72.07500000273117280, 11.83890561707634781 ) ) ;
#18909=CARTESIAN_POINT ( 'NONE',  ( -13.91746824999999887, 81.37500000273118417, 0.000000000000000000 ) ) ;
#18913=CARTESIAN_POINT ( 'NONE',  ( 9.527563637176564626, 74.00000000000000000, 10.15519155137115881 ) ) ;
#18938=CARTESIAN_POINT ( 'NONE',  ( -8.601468415847515203, 79.17500000273116711, 11.83890561707634959 ) ) ;
#18993=CARTESIAN_POINT ( 'NONE',  ( 12.13525491562420910, 75.45000000546237118, -8.816778784387098611 ) ) ;
#19008=CARTESIAN_POINT ( 'NONE',  ( 4.635254915624212657, 70.85000000546237686, 14.26584774442730286 ) ) ;
#19017=( BOUNDED_CURVE ( )  B_SPLINE_CURVE ( 2, ( #15371, #7288, #12446, #2665, #22916, #31309, #18292, #17773, #28564, #2316, #5060, #15197, #28737 ),
 .UNSPECIFIED., .F., .T. ) 
 B_SPLINE_CURVE_WITH_KNOTS ( ( 3, 2, 2, 2, 2, 2, 3 ),
 ( 0.05000000000000000278, 0.05999999999999999778, 0.08000000000000000167, 0.1000000000000000056, 0.1199999999999999956, 0.1400000000000000133, 0.1500000000000000222 ),
 .UNSPECIFIED. ) 
 CURVE ( )  GEOMETRIC_REPRESENTATION_ITEM ( )  RATIONAL_B_SPLINE_CURVE ( ( 0.9755282581475768211, 0.9755282581475768211, 1.000000000000000000, 0.9510565162951535312, 1.000000000000000000, 0.9510565162951535312, 1.000000000000000000, 0.9510565162951535312, 1.000000000000000000, 0.9510565162951535312, 1.000000000000000000, 0.9755282581475767101, 0.9755282581475768211 ) ) 
 REPRESENTATION_ITEM ( '' )  );
#19075=CARTESIAN_POINT ( 'NONE',  ( 13.91746824999999532, 78.47500000273120691, -4.522059556121118540 ) ) ;
#19140=LINE ( 'NONE', #13983, #8535 ) ;
#19151=VERTEX_POINT ( 'NONE', #13359 ) ;
#19166=CARTESIAN_POINT ( 'NONE',  ( 2.375766604868040144, 76.80125428700922896, 15.00000000000000178 ) ) ;
#19170=DIRECTION ( 'NONE',  ( 0.000000000000000000, 1.000000000000000000, 0.000000000000000000 ) ) ;
#19174=CARTESIAN_POINT ( 'NONE',  ( -8.601468415847515203, 73.17500000273119554, 11.83890561707634959 ) ) ;
#19179=CARTESIAN_POINT ( 'NONE',  ( 1.102182119232617911E-15, 74.00000000000001421, 9.000000000000001776 ) ) ;
#19220=CYLINDRICAL_SURFACE ( 'NONE', #11653, 15.00000000000000000 ) ;
#19226=CARTESIAN_POINT ( 'NONE',  ( -8.601468415847518756, 73.07500000273118701, -11.83890561707634781 ) ) ;
#19239=CARTESIAN_POINT ( 'NONE',  ( 8.601468415847516980, 78.67500000273119554, -11.83890561707634781 ) ) ;
#19246=DIRECTION ( 'NONE',  ( 0.000000000000000000, -1.000000000000000000, 0.000000000000000000 ) ) ;
#19247=CARTESIAN_POINT ( 'NONE',  ( 2.688165632520823219E-15, 77.87500000273119838, 14.63369212191046209 ) ) ;
#19263=CARTESIAN_POINT ( 'NONE',  ( -8.601468415847518756, 80.57500000273118701, -11.83890561707634781 ) ) ;
#19302=EDGE_CURVE ( 'NONE', #25891, #10457, #17672, .T. ) ;
#19310=ORIENTED_EDGE ( 'NONE', *, *, #7949, .T. ) ;
#19336=CARTESIAN_POINT ( 'NONE',  ( 2.688165632520823219E-15, 73.37500000273118417, 14.63369212191046387 ) ) ;
#19392=CARTESIAN_POINT ( 'NONE',  ( 4.300734207923761154, 71.97500000273122112, 13.23629886949340495 ) ) ;
#19406=CARTESIAN_POINT ( 'NONE',  ( -13.91746824999999532, 73.27500000273118985, -4.522059556121115875 ) ) ;
#19415=CARTESIAN_POINT ( 'NONE',  ( -4.300734207923755825, 79.77500000273118985, 13.23629886949340673 ) ) ;
#19430=( GEOMETRIC_REPRESENTATION_CONTEXT ( 3 ) GLOBAL_UNCERTAINTY_ASSIGNED_CONTEXT ( ( #18885 ) ) GLOBAL_UNIT_ASSIGNED_CONTEXT ( ( #6321, #22281, #1320 ) ) REPRESENTATION_CONTEXT ( 'NONE', 'WORKASPACE' ) );
#19431=CARTESIAN_POINT ( 'NONE',  ( -11.25946833292375793, 78.67500000273119554, -8.180482586598733619 ) ) ;
#19476=AXIS2_PLACEMENT_3D ( 'NONE', #1822, #2000, #33576 ) ;
#19485=ORIENTED_EDGE ( 'NONE', *, *, #17210, .T. ) ;
#19488=CARTESIAN_POINT ( 'NONE',  ( 9.270509831248421762, 75.55000000546240813, -12.75976212528059861 ) ) ;
#19503=( BOUNDED_CURVE ( )  B_SPLINE_CURVE ( 2, ( #11562, #24608, #23187, #33649, #10146, #16894, #27357 ),
 .UNSPECIFIED., .F., .T. ) 
 B_SPLINE_CURVE_WITH_KNOTS ( ( 3, 2, 2, 3 ),
 ( 0.000000000000000000, 0.02000000000000000042, 0.04000000000000000083, 0.05000000000000000971 ),
 .UNSPECIFIED. ) 
 CURVE ( )  GEOMETRIC_REPRESENTATION_ITEM ( )  RATIONAL_B_SPLINE_CURVE ( ( 1.000000000000000000, 0.9510565162951535312, 1.000000000000000000, 0.9510565162951535312, 1.000000000000000000, 0.9755282581475768211, 0.9755282581475768211 ) ) 
 REPRESENTATION_ITEM ( '' )  );
#19505=CARTESIAN_POINT ( 'NONE',  ( 13.91746824999999887, 77.87500000273116996, -1.704398294459741270E-15 ) ) ;
#19574=CARTESIAN_POINT ( 'NONE',  ( -11.25946833292375793, 71.57500000273120122, 8.180482586598737171 ) ) ;
#19583=CARTESIAN_POINT ( 'NONE',  ( 4.300734207923761154, 77.97500000273122112, 13.23629886949340495 ) ) ;
#19608=VERTEX_POINT ( 'NONE', #11123 ) ;
#19634=ADVANCED_FACE ( 'NONE', ( #16443 ), #26895, .T. ) ;
#19639=SURFACE_STYLE_USAGE ( .BOTH. , #9156 ) ;
#19669=CARTESIAN_POINT ( 'NONE',  ( -8.960552108402742093E-16, 72.37500000273115575, -14.63369212191046387 ) ) ;
#19699=LINE ( 'NONE', #9381, #30171 ) ;
#19717=LINE ( 'NONE', #30164, #32996 ) ;
#19726=EDGE_CURVE ( 'NONE', #28806, #9414, #8568, .T. ) ;
#19739=CARTESIAN_POINT ( 'NONE',  ( -13.91746824999999532, 75.27500000273118985, -4.522059556121115875 ) ) ;
#19748=CARTESIAN_POINT ( 'NONE',  ( 8.601468415847516980, 80.67500000273118133, -11.83890561707634603 ) ) ;
#19750=CARTESIAN_POINT ( 'NONE',  ( -15.00000000000000000, 76.15000000546238823, -4.873795443493594171 ) ) ;
#19754=CARTESIAN_POINT ( 'NONE',  ( -12.13525491562420910, 74.45000000546237118, 8.816778784387098611 ) ) ;
#19762=CARTESIAN_POINT ( 'NONE',  ( 13.91746824999999887, 71.87500000273122680, -1.704398294459741270E-15 ) ) ;
#19772=ORIENTED_EDGE ( 'NONE', *, *, #28858, .T. ) ;
#19791=VECTOR ( 'NONE', #10301, 1000.000000000000000 ) ;
#19801=VECTOR ( 'NONE', #12658, 1000.000000000000000 ) ;
#19823=CARTESIAN_POINT ( 'NONE',  ( 0.000000000000000000, 122.0000000000000000, 0.000000000000000000 ) ) ;
#19832=CARTESIAN_POINT ( 'NONE',  ( -13.91746824999999532, 72.97500000273120691, 4.522059556121122093 ) ) ;
#19863=CARTESIAN_POINT ( 'NONE',  ( -14.09332452378496470, 74.00000000000002842, 4.636822204800125746 ) ) ;
#19884=CARTESIAN_POINT ( 'NONE',  ( -4.223320258572821363E-15, 78.75000000546236834, 15.00000000000000355 ) ) ;
#19907=CARTESIAN_POINT ( 'NONE',  ( 4.300734207923761154, 71.97500000273122112, 13.23629886949340495 ) ) ;
#19918=CARTESIAN_POINT ( 'NONE',  ( -8.601468415847515203, 77.67500000273122396, 11.83890561707634959 ) ) ;
#19920=CARTESIAN_POINT ( 'NONE',  ( -15.00000000000000000, 78.35000000546239107, 4.873795443493597723 ) ) ;
#19933=CARTESIAN_POINT ( 'NONE',  ( -11.25946833292375793, 71.07500000273120122, 8.180482586598737171 ) ) ;
#19944=VECTOR ( 'NONE', #9481, 1000.000000000000000 ) ;
#19987=ORIENTED_EDGE ( 'NONE', *, *, #15988, .F. ) ;
#19993=CARTESIAN_POINT ( 'NONE',  ( -2.375766604868041476, 76.44874571845316780, 14.99999999999999822 ) ) ;
#20040=CARTESIAN_POINT ( 'NONE',  ( -5.609029516820829286, 74.00000000000004263, 13.21632355367902711 ) ) ;
#20072=EDGE_CURVE ( 'NONE', #4440, #871, #1724, .T. ) ;
#20076=ORIENTED_EDGE ( 'NONE', *, *, #2221, .T. ) ;
#20085=CARTESIAN_POINT ( 'NONE',  ( -4.635254915624211769, 81.60000000000000853, -14.26584774442730286 ) ) ;
#20096=CARTESIAN_POINT ( 'NONE',  ( -12.13525491562421088, 78.05000000546242234, -8.816778784387096835 ) ) ;
#20109=CARTESIAN_POINT ( 'NONE',  ( -8.601468415847518756, 74.57500000273120122, -11.83890561707634781 ) ) ;
#20139=CIRCLE ( 'NONE', #13012, 9.000000000000001776 ) ;
#20183=CARTESIAN_POINT ( 'NONE',  ( -11.25946833292375793, 71.07500000273120122, 8.180482586598737171 ) ) ;
#20194=CARTESIAN_POINT ( 'NONE',  ( -4.635254915624208216, 78.39999999999996305, 14.26584774442730463 ) ) ;
#20203=EDGE_CURVE ( 'NONE', #18278, #10457, #28673, .T. ) ;
#20205=( BOUNDED_CURVE ( )  B_SPLINE_CURVE ( 2, ( #24772, #1250, #9153, #30552, #17530, #14954, #1898, #29165, #5502, #24038, #8234, #18557, #20796, #163, #2594, #10653, #21303, #2419, #15982, #18388, #10483, #28497, #29001, #18222, #10823, #31907, #3104, #2930, #7732, #13222, #26438, #20961, #18728, #10992, #507, #28668, #13400, #28834, #21131, #15813, #31573, #23870, #5161, #23697, #338, #31411, #5673, #21465, #8402, #15646, #31743, #5332, #8071, #26268, #16153, #2756, #33823, #23362, #26606, #12886, #13575, #25925, #13057, #18890, #4990, #15472, #10317, #31240, #26097, #23530, #7904 ),
 .UNSPECIFIED., .F., .T. ) 
 B_SPLINE_CURVE_WITH_KNOTS ( ( 3, 2, 2, 2, 2, 2, 2, 2, 2, 2, 2, 2, 2, 2, 2, 2, 2, 2, 2, 2, 2, 2, 2, 2, 2, 2, 2, 2, 2, 2, 2, 2, 2, 2, 2, 3 ),
 ( 0.000000000000000000, 0.02000000000000000042, 0.04000000000000000083, 0.05999999999999999778, 0.08000000000000000167, 0.1000000000000000056, 0.1199999999999999956, 0.1400000000000000133, 0.1600000000000000033, 0.1799999999999999933, 0.2000000000000000111, 0.2200000000000000289, 0.2399999999999999911, 0.2600000000000000089, 0.2800000000000000266, 0.2999999999999999889, 0.3200000000000000067, 0.3400000000000000244, 0.3599999999999999867, 0.3800000000000000044, 0.4000000000000000222, 0.4200000000000000400, 0.4400000000000000577, 0.4600000000000000755, 0.4799999999999999822, 0.5000000000000000000, 0.5200000000000000178, 0.5400000000000000355, 0.5600000000000000533, 0.5799999999999999600, 0.5999999999999999778, 0.6199999999999999956, 0.6400000000000000133, 0.6600000000000000311, 0.6800000000000000488, 0.6875575298689673431 ),
 .UNSPECIFIED. ) 
 CURVE ( )  GEOMETRIC_REPRESENTATION_ITEM ( )  RATIONAL_B_SPLINE_CURVE ( ( 1.000000000000000000, 0.9510565162951535312, 1.000000000000000000, 0.9510565162951535312, 1.000000000000000000, 0.9510565162951535312, 1.000000000000000000, 0.9510565162951535312, 1.000000000000000000, 0.9510565162951535312, 1.000000000000000000, 0.9510565162951535312, 1.000000000000000000, 0.9510565162951535312, 1.000000000000000000, 0.9510565162951535312, 1.000000000000000000, 0.9510565162951535312, 1.000000000000000000, 0.9510565162951535312, 1.000000000000000000, 0.9510565162951535312, 1.000000000000000000, 0.9510565162951535312, 1.000000000000000000, 0.9510565162951535312, 1.000000000000000000, 0.9510565162951535312, 1.000000000000000000, 0.9510565162951535312, 1.000000000000000000, 0.9510565162951535312, 1.000000000000000000, 0.9510565162951535312, 1.000000000000000000, 0.9510565162951535312, 1.000000000000000000, 0.9510565162951535312, 1.000000000000000000, 0.9510565162951535312, 1.000000000000000000, 0.9510565162951535312, 1.000000000000000000, 0.9510565162951535312, 1.000000000000000000, 0.9510565162951535312, 1.000000000000000000, 0.9510565162951535312, 1.000000000000000000, 0.9510565162951535312, 1.000000000000000000, 0.9510565162951535312, 1.000000000000000000, 0.9510565162951535312, 1.000000000000000000, 0.9510565162951535312, 1.000000000000000000, 0.9510565162951535312, 1.000000000000000000, 0.9510565162951535312, 1.000000000000000000, 0.9510565162951535312, 1.000000000000000000, 0.9510565162951535312, 1.000000000000000000, 0.9510565162951535312, 1.000000000000000000, 0.9510565162951535312, 1.000000000000000000, 0.9815054080004653736, 0.9769881591460154446 ) ) 
 REPRESENTATION_ITEM ( '' )  );
#20209=FACE_OUTER_BOUND ( 'NONE', #5300, .T. ) ;
#20217=CARTESIAN_POINT ( 'NONE',  ( -10.57675453070074312, 74.00000000000000000, 10.05591069532431625 ) ) ;
#20231=CARTESIAN_POINT ( 'NONE',  ( 23.09401076758502569, 96.00000000000002842, -6.857326241137392698E-15 ) ) ;
#20238=CARTESIAN_POINT ( 'NONE',  ( -12.13525491562421088, 78.05000000546242234, -8.816778784387096835 ) ) ;
#20257=CARTESIAN_POINT ( 'NONE',  ( -4.635254915624211769, 79.60000000000000853, -14.26584774442730286 ) ) ;
#20267=CARTESIAN_POINT ( 'NONE',  ( -12.13525491562421088, 76.05000000546240813, -8.816778784387096835 ) ) ;
#20272=CARTESIAN_POINT ( 'NONE',  ( -15.00000000000000000, 74.25000000546239676, 0.000000000000000000 ) ) ;
#20280=CARTESIAN_POINT ( 'NONE',  ( 11.25946833292375793, 73.67500000273119554, 8.180482586598731842 ) ) ;
#20288=ORIENTED_EDGE ( 'NONE', *, *, #18079, .F. ) ;
#20293=ORIENTED_EDGE ( 'NONE', *, *, #2822, .T. ) ;
#20326=DIRECTION ( 'NONE',  ( 0.000000000000000000, -1.000000000000000000, 0.000000000000000000 ) ) ;
#20327=ORIENTED_EDGE ( 'NONE', *, *, #14116, .T. ) ;
#20329=FACE_OUTER_BOUND ( 'NONE', #1950, .T. ) ;
#20353=CARTESIAN_POINT ( 'NONE',  ( 9.270509831248421762, 75.30000000000001137, -12.75976212528059861 ) ) ;
#20383=FACE_BOUND ( 'NONE', #16348, .T. ) ;
#20412=ORIENTED_EDGE ( 'NONE', *, *, #7128, .T. ) ;
#20426=CARTESIAN_POINT ( 'NONE',  ( -12.13525491562421088, 77.80000000000003979, -8.816778784387096835 ) ) ;
#20438=CARTESIAN_POINT ( 'NONE',  ( -12.13525491562421088, 74.05000000546240813, -8.816778784387096835 ) ) ;
#20452=CARTESIAN_POINT ( 'NONE',  ( 8.601468415847520532, 75.57500000273117280, 11.83890561707634781 ) ) ;
#20457=CARTESIAN_POINT ( 'NONE',  ( 12.13525491562420910, 79.19999999999998863, -8.816778784387098611 ) ) ;
#20460=ORIENTED_EDGE ( 'NONE', *, *, #24249, .F. ) ;
#20518=( BOUNDED_CURVE ( )  B_SPLINE_CURVE ( 2, ( #32365, #797, #31864, #16439, #27056, #13529, #8859 ),
 .UNSPECIFIED., .F., .F. ) 
 B_SPLINE_CURVE_WITH_KNOTS ( ( 3, 2, 2, 3 ),
 ( 0.000000000000000000, 0.02000000000000000042, 0.04000000000000000083, 0.05000000000000000971 ),
 .UNSPECIFIED. ) 
 CURVE ( )  GEOMETRIC_REPRESENTATION_ITEM ( )  RATIONAL_B_SPLINE_CURVE ( ( 1.000000000000000000, 0.9510565162951535312, 1.000000000000000000, 0.9510565162951535312, 1.000000000000000000, 0.9755282581475768211, 0.9755282581475768211 ) ) 
 REPRESENTATION_ITEM ( '' )  );
#20522=( BOUNDED_CURVE ( )  B_SPLINE_CURVE ( 2, ( #14857, #31152, #15204, #20353, #22923, #23441, #17780, #30627, #28408, #23270, #15379, #33379, #10230 ),
 .UNSPECIFIED., .F., .T. ) 
 B_SPLINE_CURVE_WITH_KNOTS ( ( 3, 2, 2, 2, 2, 2, 3 ),
 ( 0.6500000000000000222, 0.6600000000000000311, 0.6800000000000000488, 0.6999999999999999556, 0.7199999999999999734, 0.7399999999999999911, 0.7500000000000000000 ),
 .UNSPECIFIED. ) 
 CURVE ( )  GEOMETRIC_REPRESENTATION_ITEM ( )  RATIONAL_B_SPLINE_CURVE ( ( 0.9755282581475768211, 0.9755282581475768211, 1.000000000000000000, 0.9510565162951535312, 1.000000000000000000, 0.9510565162951535312, 1.000000000000000000, 0.9510565162951535312, 1.000000000000000000, 0.9510565162951535312, 1.000000000000000000, 0.9755282581475768211, 0.9755282581475768211 ) ) 
 REPRESENTATION_ITEM ( '' )  );
#20548=EDGE_LOOP ( 'NONE', ( #27838, #28632, #28344, #19772, #19485, #15309, #30434, #30475, #23156, #18782, #27405, #22551 ) ) ;
#20584=DIRECTION ( 'NONE',  ( 0.000000000000000000, 1.000000000000000000, 0.000000000000000000 ) ) ;
#20607=CARTESIAN_POINT ( 'NONE',  ( -15.00000000000000000, 77.89999999999999147, -4.873795443493594171 ) ) ;
#20631=CARTESIAN_POINT ( 'NONE',  ( 2.688165632520823219E-15, 79.87500000273114154, 14.63369212191046387 ) ) ;
#20645=EDGE_CURVE ( 'NONE', #22878, #17411, #22397, .T. ) ;
#20710=CARTESIAN_POINT ( 'NONE',  ( -4.300734207923755825, 71.27500000273117564, 13.23629886949340673 ) ) ;
#20730=CARTESIAN_POINT ( 'NONE',  ( 0.000000000000000000, 102.0000000000000284, 0.000000000000000000 ) ) ;
#20759=CARTESIAN_POINT ( 'NONE',  ( 0.000000000000000000, 111.9999999999999858, 0.000000000000000000 ) ) ;
#20775=CARTESIAN_POINT ( 'NONE',  ( 15.00000000000000000, 75.10000000000002274, -4.873795443493596835 ) ) ;
#20788=CARTESIAN_POINT ( 'NONE',  ( -14.45873412499999944, 81.68750000136559208, 0.000000000000000000 ) ) ;
#20796=CARTESIAN_POINT ( 'NONE',  ( 11.25946833292375793, 79.67500000273119554, 8.180482586598731842 ) ) ;
#20799=CARTESIAN_POINT ( 'NONE',  ( 4.300734207923761154, 75.97500000273122112, 13.23629886949340495 ) ) ;
#20845=VERTEX_POINT ( 'NONE', #31929 ) ;
#20940=CARTESIAN_POINT ( 'NONE',  ( -9.657523855033125146E-16, 77.50000000000000000, -15.77193336357400710 ) ) ;
#20961=CARTESIAN_POINT ( 'NONE',  ( 13.91746825000000065, 77.77500000273116143, 4.522059556121115875 ) ) ;
#20964=CARTESIAN_POINT ( 'NONE',  ( -8.601468415847515203, 79.67500000273115290, 11.83890561707634959 ) ) ;
#20976=LINE ( 'NONE', #9, #23991 ) ;
#20982=CARTESIAN_POINT ( 'NONE',  ( -9.270509831248419985, 76.55000000546239391, 12.75976212528060039 ) ) ;
#20984=CARTESIAN_POINT ( 'NONE',  ( 13.18564821210877014, 74.00000000000005684, 4.476740745196889470 ) ) ;
#20994=LINE ( 'NONE', #2626, #12949 ) ;
#21082=CARTESIAN_POINT ( 'NONE',  ( -4.635254915624211769, 73.85000000546237686, -14.26584774442730286 ) ) ;
#21100=ORIENTED_EDGE ( 'NONE', *, *, #26669, .T. ) ;
#21131=CARTESIAN_POINT ( 'NONE',  ( -11.25946833292375793, 77.07500000273121543, 8.180482586598737171 ) ) ;
#21135=CARTESIAN_POINT ( 'NONE',  ( 13.91746824999999532, 74.47500000273120691, -4.522059556121118540 ) ) ;
#21150=CARTESIAN_POINT ( 'NONE',  ( 4.300734207923757602, 76.77500000273118985, -13.23629886949340673 ) ) ;
#21185=CARTESIAN_POINT ( 'NONE',  ( 4.635254915624209993, 77.39999999999996305, -14.26584774442730463 ) ) ;
#21200=CARTESIAN_POINT ( 'NONE',  ( -15.00000000000000000, 74.00000000000001421, 0.000000000000000000 ) ) ;
#21230=CARTESIAN_POINT ( 'NONE',  ( 0.000000000000000000, 122.0000000000000000, 0.000000000000000000 ) ) ;
#21252=CARTESIAN_POINT ( 'NONE',  ( -4.300734207923759378, 80.47500000273116427, -13.23629886949340495 ) ) ;
#21264=EDGE_CURVE ( 'NONE', #4440, #28702, #33971, .T. ) ;
#21292=CARTESIAN_POINT ( 'NONE',  ( -2.111130048464370024, 74.00000000000002842, -14.50686135258029630 ) ) ;
#21295=DIRECTION ( 'NONE',  ( 0.000000000000000000, -0.000000000000000000, 1.000000000000000000 ) ) ;
#21302=DIRECTION ( 'NONE',  ( -0.8660254037844388186, 0.000000000000000000, -0.4999999999999996669 ) ) ;
#21303=CARTESIAN_POINT ( 'NONE',  ( -4.300734207923755825, 79.27500000273118985, 13.23629886949340673 ) ) ;
#21306=CARTESIAN_POINT ( 'NONE',  ( 11.25946833292375793, 74.17500000273119554, 8.180482586598731842 ) ) ;
#21319=CARTESIAN_POINT ( 'NONE',  ( 13.91746825000000065, 76.27500000273116143, 4.522059556121114987 ) ) ;
#21394=ORIENTED_EDGE ( 'NONE', *, *, #28858, .F. ) ;
#21416=CARTESIAN_POINT ( 'NONE',  ( -15.00000000000000000, 72.15000000546238823, -4.873795443493594171 ) ) ;
#21463=AXIS2_PLACEMENT_3D ( 'NONE', #21230, #27201, #3692 ) ;
#21465=CARTESIAN_POINT ( 'NONE',  ( 8.601468415847516980, 76.17500000273116711, -11.83890561707634603 ) ) ;
#21480=CARTESIAN_POINT ( 'NONE',  ( 13.91746825000000065, 78.27500000273118985, 4.522059556121114987 ) ) ;
#21493=CARTESIAN_POINT ( 'NONE',  ( 5.348221797398307942, 74.00000000000001421, 12.84883053416113974 ) ) ;
#21496=CARTESIAN_POINT ( 'NONE',  ( 0.000000000000000000, 111.9999999999999858, 0.000000000000000000 ) ) ;
#21505=CARTESIAN_POINT ( 'NONE',  ( 4.300734207923757602, 76.27500000273118985, -13.23629886949340673 ) ) ;
#21552=EDGE_CURVE ( 'NONE', #11228, #4064, #31293, .T. ) ;
#21581=CARTESIAN_POINT ( 'NONE',  ( -15.00000000000000000, 72.35000000546239107, 4.873795443493597723 ) ) ;
#21605=ORIENTED_EDGE ( 'NONE', *, *, #15946, .T. ) ;
#21665=DIRECTION ( 'NONE',  ( 0.000000000000000000, 0.000000000000000000, 1.000000000000000000 ) ) ;
#21673=CARTESIAN_POINT ( 'NONE',  ( -11.25946833292375793, 76.67500000273119554, -8.180482586598733619 ) ) ;
#21679=EDGE_CURVE ( 'NONE', #26497, #4231, #2076, .T. ) ;
#21690=DIRECTION ( 'NONE',  ( 0.8660254037844410391, 0.4999999999999958367, 0.000000000000000000 ) ) ;
#21702=CARTESIAN_POINT ( 'NONE',  ( 1.836970198721029589E-15, 74.00000000000001421, -15.00000000000000000 ) ) ;
#21704=ORIENTED_EDGE ( 'NONE', *, *, #3277, .T. ) ;
#21746=EDGE_CURVE ( 'NONE', #18703, #8542, #19699, .T. ) ;
#21751=CARTESIAN_POINT ( 'NONE',  ( -9.657523855033125146E-16, 71.75000000546242518, -15.77193336357400710 ) ) ;
#21759=CARTESIAN_POINT ( 'NONE',  ( -2.375766604868045029, 79.55125428154684641, -14.99999999999999822 ) ) ;
#21781=DIRECTION ( 'NONE',  ( 0.000000000000000000, 0.000000000000000000, 1.000000000000000000 ) ) ;
#21792=CARTESIAN_POINT ( 'NONE',  ( -13.91746824999999887, 81.37500000273118417, 0.000000000000000000 ) ) ;
#21814=CARTESIAN_POINT ( 'NONE',  ( -4.300734207923759378, 78.97500000273122112, -13.23629886949340495 ) ) ;
#21818=DIRECTION ( 'NONE',  ( 1.000000000000000000, 0.000000000000000000, 0.000000000000000000 ) ) ;
#21833=FACE_OUTER_BOUND ( 'NONE', #15052, .T. ) ;
#21841=CARTESIAN_POINT ( 'NONE',  ( 8.601468415847520532, 79.57500000273117280, 11.83890561707634781 ) ) ;
#21910=CARTESIAN_POINT ( 'NONE',  ( -4.300734207923755825, 75.27500000273118985, 13.23629886949340673 ) ) ;
#21916=CARTESIAN_POINT ( 'NONE',  ( -8.891200544363830713E-16, 79.49999999999998579, -15.00000000000000000 ) ) ;
#21926=VERTEX_POINT ( 'NONE', #7505 ) ;
#21957=UNCERTAINTY_MEASURE_WITH_UNIT (LENGTH_MEASURE( 1.000000000000000082E-05 ), #13404, 'distance_accuracy_value', 'NONE');
#21964=DIRECTION ( 'NONE',  ( 0.000000000000000000, 0.000000000000000000, 1.000000000000000000 ) ) ;
#21978=CARTESIAN_POINT ( 'NONE',  ( 12.13525491562420910, 81.19999999999998863, -8.816778784387098611 ) ) ;
#21988=CARTESIAN_POINT ( 'NONE',  ( 13.91746824999999887, 80.37500000273118417, -1.704398294459741270E-15 ) ) ;
#21995=LINE ( 'NONE', #8944, #23958 ) ;
#22004=CARTESIAN_POINT ( 'NONE',  ( 13.91746824999999887, 77.87500000273116996, -1.704398294459741270E-15 ) ) ;
#22011=CARTESIAN_POINT ( 'NONE',  ( 2.445080149700053643E-15, 76.50000000000001421, 15.00000000000000000 ) ) ;
#22018=VERTEX_POINT ( 'NONE', #28436 ) ;
#22079=CARTESIAN_POINT ( 'NONE',  ( 4.300734207923757602, 74.27500000273118985, -13.23629886949340673 ) ) ;
#22083=VECTOR ( 'NONE', #31104, 1000.000000000000000 ) ;
#22086=CARTESIAN_POINT ( 'NONE',  ( -9.270509831248423538, 79.69999999999997442, -12.75976212528059861 ) ) ;
#22149=CARTESIAN_POINT ( 'NONE',  ( -11.25946833292375793, 73.17500000273119554, -8.180482586598733619 ) ) ;
#22160=CARTESIAN_POINT ( 'NONE',  ( 11.25946833292375793, 76.57500000273120122, -8.180482586598735395 ) ) ;
#22175=CARTESIAN_POINT ( 'NONE',  ( -11.25946833292375793, 77.07500000273121543, 8.180482586598737171 ) ) ;
#22214=SURFACE_STYLE_FILL_AREA ( #1253 ) ;
#22231=VECTOR ( 'NONE', #759, 1000.000000000000000 ) ;
#22246=CARTESIAN_POINT ( 'NONE',  ( -13.91746824999999532, 74.97500000273117848, 4.522059556121122093 ) ) ;
#22263=ORIENTED_EDGE ( 'NONE', *, *, #3157, .T. ) ;
#22275=DIRECTION ( 'NONE',  ( 0.000000000000000000, 0.000000000000000000, 1.000000000000000000 ) ) ;
#22276=CARTESIAN_POINT ( 'NONE',  ( -9.225643108219712119, 73.99999999999998579, 11.22019004876342763 ) ) ;
#22281=( NAMED_UNIT ( * ) PLANE_ANGLE_UNIT ( ) SI_UNIT ( $, .RADIAN. ) );
#22296=CARTESIAN_POINT ( 'NONE',  ( -4.635254915624211769, 77.85000000546237686, -14.26584774442730286 ) ) ;
#22315=CARTESIAN_POINT ( 'NONE',  ( -4.300734207923759378, 74.97500000273122112, -13.23629886949340495 ) ) ;
#22325=CARTESIAN_POINT ( 'NONE',  ( 4.300734207923757602, 78.77500000273118985, -13.23629886949340673 ) ) ;
#22327=CARTESIAN_POINT ( 'NONE',  ( 12.13525491562420910, 77.45000000546237118, -8.816778784387098611 ) ) ;
#22339=CARTESIAN_POINT ( 'NONE',  ( 13.91746825000000065, 75.77500000273117564, 4.522059556121114987 ) ) ;
#22366=CARTESIAN_POINT ( 'NONE',  ( -11.54700538379251995, 96.00000000000002842, -19.99999999999999645 ) ) ;
#22368=EDGE_CURVE ( 'NONE', #21926, #22878, #24797, .T. ) ;
#22387=CARTESIAN_POINT ( 'NONE',  ( -9.270509831248419985, 74.29999999999999716, 12.75976212528060039 ) ) ;
#22391=CARTESIAN_POINT ( 'NONE',  ( 2.445080149700053643E-15, 76.50000000000001421, 15.00000000000000000 ) ) ;
#22397=( BOUNDED_CURVE ( )  B_SPLINE_CURVE ( 2, ( #23552, #5693, #2440, #20982, #18066, #29021, #16002, #26458, #31260, #16171, #23382, #29188, #7754 ),
 .UNSPECIFIED., .F., .T. ) 
 B_SPLINE_CURVE_WITH_KNOTS ( ( 3, 2, 2, 2, 2, 2, 3 ),
 ( 0.3500000000000000333, 0.3599999999999999867, 0.3800000000000000044, 0.4000000000000000222, 0.4199999999999999845, 0.4400000000000000022, 0.4500000000000000111 ),
 .UNSPECIFIED. ) 
 CURVE ( )  GEOMETRIC_REPRESENTATION_ITEM ( )  RATIONAL_B_SPLINE_CURVE ( ( 0.9755282581475768211, 0.9755282581475768211, 1.000000000000000000, 0.9510565162951535312, 1.000000000000000000, 0.9510565162951535312, 1.000000000000000000, 0.9510565162951535312, 1.000000000000000000, 0.9510565162951535312, 1.000000000000000000, 0.9755282581475768211, 0.9755282581475768211 ) ) 
 REPRESENTATION_ITEM ( '' )  );
#22406=CARTESIAN_POINT ( 'NONE',  ( 11.25946833292375793, 78.07500000273121543, -8.180482586598735395 ) ) ;
#22435=CARTESIAN_POINT ( 'NONE',  ( -5.331399199010175671, 74.00000000000000000, 13.31861229302914928 ) ) ;
#22453=CARTESIAN_POINT ( 'NONE',  ( -8.891200544363830713E-16, 77.75000000546235412, -15.00000000000000000 ) ) ;
#22475=CARTESIAN_POINT ( 'NONE',  ( -8.601468415847518756, 75.07500000273118701, -11.83890561707634781 ) ) ;
#22484=CARTESIAN_POINT ( 'NONE',  ( 11.25946833292375793, 76.17500000273119554, 8.180482586598731842 ) ) ;
#22486=CARTESIAN_POINT ( 'NONE',  ( -4.635254915624211769, 79.85000000546239107, -14.26584774442730286 ) ) ;
#22498=CARTESIAN_POINT ( 'NONE',  ( -13.91746824999999887, 81.37500000273118417, 0.000000000000000000 ) ) ;
#22520=CARTESIAN_POINT ( 'NONE',  ( 4.635254915624209993, 77.65000000546234560, -14.26584774442730463 ) ) ;
#22528=EDGE_LOOP ( 'NONE', ( #18759, #16481, #33218, #16451 ) ) ;
#22548=ORIENTED_EDGE ( 'NONE', *, *, #14116, .F. ) ;
#22551=ORIENTED_EDGE ( 'NONE', *, *, #21679, .F. ) ;
#22573=CARTESIAN_POINT ( 'NONE',  ( -8.601468415847518756, 72.57500000273114438, -11.83890561707634781 ) ) ;
#22593=EDGE_LOOP ( 'NONE', ( #29884, #27527, #13457, #27575 ) ) ;
#22603=CARTESIAN_POINT ( 'NONE',  ( -0.3918072299880378528, 74.00000000000004263, 14.19424161045959210 ) ) ;
#22631=AXIS2_PLACEMENT_3D ( 'NONE', #8742, #32080, #21964 ) ;
#22639=CARTESIAN_POINT ( 'NONE',  ( 0.000000000000000000, 74.00000000000001421, 0.000000000000000000 ) ) ;
#22647=CARTESIAN_POINT ( 'NONE',  ( -13.91746824999999532, 71.47500000273119269, 4.522059556121122093 ) ) ;
#22658=CARTESIAN_POINT ( 'NONE',  ( 9.270509831248423538, 75.55000000546242234, -12.75976212528059861 ) ) ;
#22673=CARTESIAN_POINT ( 'NONE',  ( -11.25946833292375793, 75.07500000273120122, 8.180482586598737171 ) ) ;
#22675=DIRECTION ( 'NONE',  ( 0.4999999999999996114, 0.000000000000000000, -0.8660254037844388186 ) ) ;
#22707=LINE ( 'NONE', #30239, #8512 ) ;
#22733=VERTEX_POINT ( 'NONE', #27849 ) ;
#22744=DIRECTION ( 'NONE',  ( 0.000000000000000000, 1.000000000000000000, 0.000000000000000000 ) ) ;
#22779=LINE ( 'NONE', #25529, #30219 ) ;
#22780=CARTESIAN_POINT ( 'NONE',  ( 3.115048150918978465, 74.00000000000002842, 13.67161610608823530 ) ) ;
#22820=CARTESIAN_POINT ( 'NONE',  ( -4.635254915624208216, 74.40000000000001990, 14.26584774442730463 ) ) ;
#22831=CARTESIAN_POINT ( 'NONE',  ( -4.635254915624208216, 78.65000000546234560, 14.26584774442730463 ) ) ;
#22846=CARTESIAN_POINT ( 'NONE',  ( -13.91746824999999532, 81.27500000273117564, -4.522059556121115875 ) ) ;
#22860=ORIENTED_EDGE ( 'NONE', *, *, #18514, .T. ) ;
#22878=VERTEX_POINT ( 'NONE', #25017 ) ;
#22894=DIRECTION ( 'NONE',  ( 0.000000000000000000, 1.000000000000000000, 0.000000000000000000 ) ) ;
#22904=EDGE_CURVE ( 'NONE', #17164, #28702, #12139, .T. ) ;
#22916=CARTESIAN_POINT ( 'NONE',  ( 12.13525491562420910, 81.19999999999998863, -8.816778784387098611 ) ) ;
#22923=CARTESIAN_POINT ( 'NONE',  ( 12.13525491562420910, 75.19999999999998863, -8.816778784387098611 ) ) ;
#22980=VERTEX_POINT ( 'NONE', #11973 ) ;
#22984=ORIENTED_EDGE ( 'NONE', *, *, #29234, .F. ) ;
#22990=CARTESIAN_POINT ( 'NONE',  ( 12.13525491562421088, 79.05000000546236549, 8.816778784387095058 ) ) ;
#22993=CARTESIAN_POINT ( 'NONE',  ( -4.635254915624211769, 75.59999999999999432, -14.26584774442730286 ) ) ;
#23006=CARTESIAN_POINT ( 'NONE',  ( -9.270509831248421762, 74.55000000546239391, 12.75976212528060039 ) ) ;
#23018=CARTESIAN_POINT ( 'NONE',  ( 0.000000000000000000, 122.0000000000000000, 10.64101615137753676 ) ) ;
#23021=CARTESIAN_POINT ( 'NONE',  ( -8.960552108402742093E-16, 74.37500000273121259, -14.63369212191046387 ) ) ;
#23079=CARTESIAN_POINT ( 'NONE',  ( 23.09401076758502569, 96.00000000000002842, -6.857326241137392698E-15 ) ) ;
#23090=AXIS2_PLACEMENT_3D ( 'NONE', #9764, #7187, #2041 ) ;
#23156=ORIENTED_EDGE ( 'NONE', *, *, #27079, .T. ) ;
#23160=CARTESIAN_POINT ( 'NONE',  ( 12.13525491562420910, 79.45000000546237118, -8.816778784387098611 ) ) ;
#23164=CARTESIAN_POINT ( 'NONE',  ( 15.00000000000000000, 79.00000000000001421, -1.836970198721029589E-15 ) ) ;
#23177=CARTESIAN_POINT ( 'NONE',  ( -11.25946833292375793, 79.07500000273121543, 8.180482586598737171 ) ) ;
#23187=CARTESIAN_POINT ( 'NONE',  ( -12.13525491562421088, 81.79999999999998295, -8.816778784387096835 ) ) ;
#23190=CARTESIAN_POINT ( 'NONE',  ( 13.91746825000000065, 74.27500000273120406, 4.522059556121114987 ) ) ;
#23218=( BOUNDED_CURVE ( )  B_SPLINE_CURVE ( 2, ( #19884, #9752, #1852, #25199, #1338, #12152, #1509, #4095, #20238, #11984, #22296, #32741, #22453 ),
 .UNSPECIFIED., .F., .T. ) 
 B_SPLINE_CURVE_WITH_KNOTS ( ( 3, 2, 2, 2, 2, 2, 3 ),
 ( 0.1500000000000000222, 0.1600000000000000033, 0.1799999999999999933, 0.2000000000000000111, 0.2200000000000000011, 0.2399999999999999911, 0.2500000000000000000 ),
 .UNSPECIFIED. ) 
 CURVE ( )  GEOMETRIC_REPRESENTATION_ITEM ( )  RATIONAL_B_SPLINE_CURVE ( ( 0.9755282581475768211, 0.9755282581475768211, 1.000000000000000000, 0.9510565162951535312, 1.000000000000000000, 0.9510565162951535312, 1.000000000000000000, 0.9510565162951535312, 1.000000000000000000, 0.9510565162951535312, 1.000000000000000000, 0.9755282581475768211, 0.9755282581475768211 ) ) 
 REPRESENTATION_ITEM ( '' )  );
#23224=DIRECTION ( 'NONE',  ( 0.000000000000000000, 0.000000000000000000, 1.000000000000000000 ) ) ;
#23263=CARTESIAN_POINT ( 'NONE',  ( -1.089172066684569321E-14, 78.49999999999998579, 15.00000000000000000 ) ) ;
#23270=CARTESIAN_POINT ( 'NONE',  ( 9.270509831248425314, 74.69999999999996021, 12.75976212528059683 ) ) ;
#23275=DIRECTION ( 'NONE',  ( 0.000000000000000000, 0.000000000000000000, -1.000000000000000000 ) ) ;
#23332=VECTOR ( 'NONE', #27244, 1000.000000000000000 ) ;
#23343=CARTESIAN_POINT ( 'NONE',  ( 15.00000000000000355, 78.90000000000001990, 4.873795443493592394 ) ) ;
#23353=CARTESIAN_POINT ( 'NONE',  ( -4.300734207923759378, 74.97500000273122112, -13.23629886949340495 ) ) ;
#23362=CARTESIAN_POINT ( 'NONE',  ( -8.601468415847515203, 75.17500000273118133, 11.83890561707634959 ) ) ;
#23365=CARTESIAN_POINT ( 'NONE',  ( 13.91746825000000065, 76.27500000273116143, 4.522059556121114987 ) ) ;
#23382=CARTESIAN_POINT ( 'NONE',  ( -4.635254915624211769, 75.85000000546237686, -14.26584774442730286 ) ) ;
#23387=CARTESIAN_POINT ( 'NONE',  ( 11.54700538379251817, 86.00000000000001421, 19.99999999999999645 ) ) ;
#23412=DIRECTION ( 'NONE',  ( 0.5000000000000000000, 0.000000000000000000, 0.8660254037844385966 ) ) ;
#23426=VECTOR ( 'NONE', #5306, 1000.000000000000000 ) ;
#23441=CARTESIAN_POINT ( 'NONE',  ( 15.00000000000000000, 75.10000000000000853, -4.873795443493596835 ) ) ;
#23468=DIRECTION ( 'NONE',  ( -0.000000000000000000, -1.000000000000000000, -0.000000000000000000 ) ) ;
#23510=CARTESIAN_POINT ( 'NONE',  ( -12.13525491562420910, 74.19999999999998863, 8.816778784387098611 ) ) ;
#23520=CARTESIAN_POINT ( 'NONE',  ( -9.688038132598597585, 73.99999999999998579, -11.40930151615730814 ) ) ;
#23530=CARTESIAN_POINT ( 'NONE',  ( 12.23270501248084585, 74.03838462613526872, -6.840937216516965513 ) ) ;
#23534=CARTESIAN_POINT ( 'NONE',  ( 8.601468415847520532, 78.07500000273120122, 11.83890561707634781 ) ) ;
#23535=( NAMED_UNIT ( * ) PLANE_ANGLE_UNIT ( ) SI_UNIT ( $, .RADIAN. ) );
#23552=CARTESIAN_POINT ( 'NONE',  ( -1.089172066684569321E-14, 76.75000000546238255, 15.00000000000000000 ) ) ;
#23554=DIRECTION ( 'NONE',  ( -0.000000000000000000, -1.000000000000000000, -0.000000000000000000 ) ) ;
#23625=VERTEX_POINT ( 'NONE', #12233 ) ;
#23633=ADVANCED_FACE ( 'NONE', ( #9144 ), #27348, .F. ) ;
#23670=EDGE_LOOP ( 'NONE', ( #4614, #5929, #20293, #11166 ) ) ;
#23684=EDGE_CURVE ( 'NONE', #13542, #18703, #22707, .T. ) ;
#23687=CARTESIAN_POINT ( 'NONE',  ( 10.89113995073883068, 73.99999999999998579, -8.941408771340327633 ) ) ;
#23696=FACE_OUTER_BOUND ( 'NONE', #22528, .T. ) ;
#23697=CARTESIAN_POINT ( 'NONE',  ( -8.601468415847518756, 76.57500000273120122, -11.83890561707634603 ) ) ;
#23700=CARTESIAN_POINT ( 'NONE',  ( -8.601468415847518756, 75.07500000273118701, -11.83890561707634781 ) ) ;
#23716=CARTESIAN_POINT ( 'NONE',  ( -4.300734207923759378, 76.97500000273122112, -13.23629886949340495 ) ) ;
#23720=CARTESIAN_POINT ( 'NONE',  ( 13.56056531762472872, 73.99999999999997158, 3.164391494949048145 ) ) ;
#23732=EDGE_CURVE ( 'NONE', #25120, #19608, #12060, .T. ) ;
#23752=CARTESIAN_POINT ( 'NONE',  ( 12.13525491562420910, 77.19999999999998863, -8.816778784387098611 ) ) ;
#23757=AXIS2_PLACEMENT_3D ( 'NONE', #20730, #25853, #17978 ) ;
#23763=DIRECTION ( 'NONE',  ( 0.000000000000000000, 0.000000000000000000, -1.000000000000000000 ) ) ;
#23775=ADVANCED_FACE ( 'NONE', ( #11895 ), #32650, .F. ) ;
#23821=CARTESIAN_POINT ( 'NONE',  ( -13.91746824999999887, 80.87500000273118417, 0.000000000000000000 ) ) ;
#23850=CARTESIAN_POINT ( 'NONE',  ( -4.635254915624208216, 72.40000000000001990, 14.26584774442730463 ) ) ;
#23866=LINE ( 'NONE', #27097, #25921 ) ;
#23870=CARTESIAN_POINT ( 'NONE',  ( -13.91746824999999532, 76.77500000273120406, -4.522059556121115875 ) ) ;
#23873=CARTESIAN_POINT ( 'NONE',  ( -8.601468415847515203, 75.67500000273116711, 11.83890561707634959 ) ) ;
#23886=CARTESIAN_POINT ( 'NONE',  ( 13.91746824999999532, 76.47500000273120691, -4.522059556121118540 ) ) ;
#23890=CARTESIAN_POINT ( 'NONE',  ( 8.487781194200618273, 74.00000000000002842, 11.03901998437955534 ) ) ;
#23900=CARTESIAN_POINT ( 'NONE',  ( 11.54700538379251817, 86.00000000000001421, 19.99999999999999645 ) ) ;
#23958=VECTOR ( 'NONE', #14270, 1000.000000000000000 ) ;
#23982=CARTESIAN_POINT ( 'NONE',  ( -13.91746824999999887, 80.87500000273118417, 0.000000000000000000 ) ) ;
#23987=CARTESIAN_POINT ( 'NONE',  ( -4.635254915624208216, 72.65000000546240244, 14.26584774442730463 ) ) ;
#23991=VECTOR ( 'NONE', #2774, 1000.000000000000000 ) ;
#23994=LINE ( 'NONE', #5961, #7439 ) ;
#24014=CARTESIAN_POINT ( 'NONE',  ( 12.13525491562420910, 73.19999999999998863, -8.816778784387098611 ) ) ;
#24018=( BOUNDED_CURVE ( )  B_SPLINE_CURVE ( 2, ( #31465, #13277, #21185, #29220, #23752, #16035, #26490, #2985, #13453, #10877, #8284, #5726, #22011 ),
 .UNSPECIFIED., .F., .T. ) 
 B_SPLINE_CURVE_WITH_KNOTS ( ( 3, 2, 2, 2, 2, 2, 3 ),
 ( 0.4500000000000000111, 0.4600000000000000200, 0.4799999999999999822, 0.5000000000000000000, 0.5200000000000000178, 0.5400000000000000355, 0.5500000000000000444 ),
 .UNSPECIFIED. ) 
 CURVE ( )  GEOMETRIC_REPRESENTATION_ITEM ( )  RATIONAL_B_SPLINE_CURVE ( ( 0.9755282581475768211, 0.9755282581475768211, 1.000000000000000000, 0.9510565162951535312, 1.000000000000000000, 0.9510565162951535312, 1.000000000000000000, 0.9510565162951535312, 1.000000000000000000, 0.9510565162951535312, 1.000000000000000000, 0.9755282581475768211, 0.9755282581475768211 ) ) 
 REPRESENTATION_ITEM ( '' )  );
#24026=CARTESIAN_POINT ( 'NONE',  ( 5.389190825954574215, 74.00000000000005684, -13.31942880713982724 ) ) ;
#24038=CARTESIAN_POINT ( 'NONE',  ( 13.91746824999999532, 79.97500000273115006, -4.522059556121118540 ) ) ;
#24055=CARTESIAN_POINT ( 'NONE',  ( -13.91746824999999887, 79.37500000273118417, 0.000000000000000000 ) ) ;
#24059=CARTESIAN_POINT ( 'NONE',  ( 13.82924054492543853, 74.00000000000001421, -1.809887360631980524 ) ) ;
#24083=CARTESIAN_POINT ( 'NONE',  ( 13.91746825000000065, 79.77500000273116143, 4.522059556121114987 ) ) ;
#24123=LINE ( 'NONE', #8491, #14455 ) ;
#24144=CARTESIAN_POINT ( 'NONE',  ( 12.13525491562421088, 77.05000000546242234, 8.816778784387095058 ) ) ;
#24152=CARTESIAN_POINT ( 'NONE',  ( -4.635254915624208216, 70.65000000546240244, 14.26584774442730463 ) ) ;
#24155=DIRECTION ( 'NONE',  ( 0.000000000000000000, 1.000000000000000000, 0.000000000000000000 ) ) ;
#24159=CARTESIAN_POINT ( 'NONE',  ( -11.54700538379251817, 86.00000000000001421, 19.99999999999999645 ) ) ;
#24168=ORIENTED_EDGE ( 'NONE', *, *, #16412, .F. ) ;
#24220=CARTESIAN_POINT ( 'NONE',  ( -8.601468415847515203, 79.67500000273115290, 11.83890561707634959 ) ) ;
#24225=CARTESIAN_POINT ( 'NONE',  ( 5.348221797398307942, 74.00000000000001421, 12.84883053416113974 ) ) ;
#24245=CARTESIAN_POINT ( 'NONE',  ( -8.601468415847518756, 76.57500000273120122, -11.83890561707634781 ) ) ;
#24249=EDGE_CURVE ( 'NONE', #5592, #5684, #26560, .T. ) ;
#24261=EDGE_LOOP ( 'NONE', ( #29088, #27158, #743, #8875 ) ) ;
#24299=ORIENTED_EDGE ( 'NONE', *, *, #21746, .F. ) ;
#24317=( BOUNDED_SURFACE ( )  B_SPLINE_SURFACE ( 1, 2, ( 
 ( #11365, #32451, #550, #19263, #8952, #27483, #16521, #16688, #8446, #13618, #32121, #24083, #29704, #21841, #6550, #13944, #1210, #18938, #883, #14113, #716, #11037, #19431, #13777, #6208, #14278, #24407, #32286, #24571, #29880, #22004, #8779, #11523, #1043, #8618, #27316, #3807, #24735, #22175, #30045, #3473, #9116, #21673, #24245, #26973, #17024, #21505, #31954, #5883, #26815, #3311, #22339, #27653, #20452, #33124, #7221, #17361, #30903, #22673, #9627, #30727, #1901, #9976, #20109, #14957, #23021, #30555, #7051, #17533, #7397, #17882, #17706, #20280, #27994, #32785, #28165, #6880, #25072, #32948, #4481, #17195, #9804, #3973, #2074, #12376, #6714, #12202, #25423, #14445, #9451, #19762, #24902, #27825, #1387, #12550, #9278, #4141, #4652, #19933, #11861, #15132 ),
 ( #22498, #22846, #14616, #33476, #30380, #1553, #1722, #33305, #25595, #4307, #12030, #30212, #14782, #25247, #18225, #20631, #26271, #20964, #7735, #28671, #18391, #26441, #31075, #15300, #4821, #26100, #31576, #18561, #28837, #13403, #8074, #7907, #10150, #23534, #25928, #18681, #10656, #25760, #5335, #5164, #33826, #2597, #29004, #15817, #5505, #28335, #28496, #166, #2760, #13225, #10322, #23365, #15986, #31243, #20799, #4993, #2933, #23873, #2422, #33652, #341, #15475, #12890, #23700, #15650, #13060, #10486, #2245, #12719, #21135, #10826, #23190, #21306, #7569, #31414, #31746, #8237, #18052, #11163, #29169, #26610, #13905, #3107, #19226, #18731, #5842, #5676, #11323, #27105, #6004, #8907, #24532, #510, #18893, #19392, #31910, #1003, #8577, #11487, #29663, #3598 ) ),
 .UNSPECIFIED., .F., .F., .T. ) 
 B_SPLINE_SURFACE_WITH_KNOTS ( ( 2, 2 ),
 ( 3, 2, 2, 2, 2, 2, 2, 2, 2, 2, 2, 2, 2, 2, 2, 2, 2, 2, 2, 2, 2, 2, 2, 2, 2, 2, 2, 2, 2, 2, 2, 2, 2, 2, 2, 2, 2, 2, 2, 2, 2, 2, 2, 2, 2, 2, 2, 2, 2, 2, 3 ),
 ( 0.000000000000000000, 1.000000000000000000 ),
 ( 0.000000000000000000, 0.02000000000000000042, 0.04000000000000000083, 0.05999999999999999778, 0.08000000000000000167, 0.1000000000000000056, 0.1199999999999999956, 0.1400000000000000133, 0.1600000000000000033, 0.1799999999999999933, 0.2000000000000000111, 0.2200000000000000011, 0.2399999999999999911, 0.2600000000000000089, 0.2800000000000000266, 0.2999999999999999889, 0.3200000000000000067, 0.3400000000000000244, 0.3599999999999999867, 0.3800000000000000044, 0.4000000000000000222, 0.4199999999999999845, 0.4400000000000000022, 0.4600000000000000200, 0.4799999999999999822, 0.5000000000000000000, 0.5200000000000000178, 0.5400000000000000355, 0.5600000000000000533, 0.5799999999999999600, 0.5999999999999999778, 0.6199999999999999956, 0.6400000000000000133, 0.6600000000000000311, 0.6800000000000000488, 0.6999999999999999556, 0.7199999999999999734, 0.7399999999999999911, 0.7600000000000000089, 0.7800000000000000266, 0.8000000000000000444, 0.8199999999999999512, 0.8399999999999999689, 0.8599999999999999867, 0.8800000000000000044, 0.9000000000000000222, 0.9200000000000000400, 0.9399999999999999467, 0.9599999999999999645, 0.9799999999999999822, 1.000000000000000000 ),
 .UNSPECIFIED. ) 
 GEOMETRIC_REPRESENTATION_ITEM ( )  RATIONAL_B_SPLINE_SURFACE ( (
 ( 1.000000000000000000, 0.9510565162951535312, 1.000000000000000000, 0.9510565162951535312, 1.000000000000000000, 0.9510565162951535312, 1.000000000000000000, 0.9510565162951535312, 1.000000000000000000, 0.9510565162951535312, 1.000000000000000000, 0.9510565162951535312, 1.000000000000000000, 0.9510565162951535312, 1.000000000000000000, 0.9510565162951535312, 1.000000000000000000, 0.9510565162951535312, 1.000000000000000000, 0.9510565162951535312, 1.000000000000000000, 0.9510565162951535312, 1.000000000000000000, 0.9510565162951535312, 1.000000000000000000, 0.9510565162951535312, 1.000000000000000000, 0.9510565162951535312, 1.000000000000000000, 0.9510565162951535312, 1.000000000000000000, 0.9510565162951535312, 1.000000000000000000, 0.9510565162951535312, 1.000000000000000000, 0.9510565162951535312, 1.000000000000000000, 0.9510565162951535312, 1.000000000000000000, 0.9510565162951535312, 1.000000000000000000, 0.9510565162951535312, 1.000000000000000000, 0.9510565162951535312, 1.000000000000000000, 0.9510565162951535312, 1.000000000000000000, 0.9510565162951535312, 1.000000000000000000, 0.9510565162951535312, 1.000000000000000000, 0.9510565162951535312, 1.000000000000000000, 0.9510565162951535312, 1.000000000000000000, 0.9510565162951535312, 1.000000000000000000, 0.9510565162951535312, 1.000000000000000000, 0.9510565162951535312, 1.000000000000000000, 0.9510565162951535312, 1.000000000000000000, 0.9510565162951535312, 1.000000000000000000, 0.9510565162951535312, 1.000000000000000000, 0.9510565162951535312, 1.000000000000000000, 0.9510565162951535312, 1.000000000000000000, 0.9510565162951535312, 1.000000000000000000, 0.9510565162951535312, 1.000000000000000000, 0.9510565162951535312, 1.000000000000000000, 0.9510565162951535312, 1.000000000000000000, 0.9510565162951535312, 1.000000000000000000, 0.9510565162951535312, 1.000000000000000000, 0.9510565162951535312, 1.000000000000000000, 0.9510565162951535312, 1.000000000000000000, 0.9510565162951535312, 1.000000000000000000, 0.9510565162951535312, 1.000000000000000000, 0.9510565162951535312, 1.000000000000000000, 0.9510565162951535312, 1.000000000000000000, 0.9510565162951535312, 1.000000000000000000, 0.9510565162951535312, 1.000000000000000000, 0.9510565162951535312, 1.000000000000000000),
 ( 1.000000000000000000, 0.9510565162951535312, 1.000000000000000000, 0.9510565162951535312, 1.000000000000000000, 0.9510565162951535312, 1.000000000000000000, 0.9510565162951535312, 1.000000000000000000, 0.9510565162951535312, 1.000000000000000000, 0.9510565162951535312, 1.000000000000000000, 0.9510565162951535312, 1.000000000000000000, 0.9510565162951535312, 1.000000000000000000, 0.9510565162951535312, 1.000000000000000000, 0.9510565162951535312, 1.000000000000000000, 0.9510565162951535312, 1.000000000000000000, 0.9510565162951535312, 1.000000000000000000, 0.9510565162951535312, 1.000000000000000000, 0.9510565162951535312, 1.000000000000000000, 0.9510565162951535312, 1.000000000000000000, 0.9510565162951535312, 1.000000000000000000, 0.9510565162951535312, 1.000000000000000000, 0.9510565162951535312, 1.000000000000000000, 0.9510565162951535312, 1.000000000000000000, 0.9510565162951535312, 1.000000000000000000, 0.9510565162951535312, 1.000000000000000000, 0.9510565162951535312, 1.000000000000000000, 0.9510565162951535312, 1.000000000000000000, 0.9510565162951535312, 1.000000000000000000, 0.9510565162951535312, 1.000000000000000000, 0.9510565162951535312, 1.000000000000000000, 0.9510565162951535312, 1.000000000000000000, 0.9510565162951535312, 1.000000000000000000, 0.9510565162951535312, 1.000000000000000000, 0.9510565162951535312, 1.000000000000000000, 0.9510565162951535312, 1.000000000000000000, 0.9510565162951535312, 1.000000000000000000, 0.9510565162951535312, 1.000000000000000000, 0.9510565162951535312, 1.000000000000000000, 0.9510565162951535312, 1.000000000000000000, 0.9510565162951535312, 1.000000000000000000, 0.9510565162951535312, 1.000000000000000000, 0.9510565162951535312, 1.000000000000000000, 0.9510565162951535312, 1.000000000000000000, 0.9510565162951535312, 1.000000000000000000, 0.9510565162951535312, 1.000000000000000000, 0.9510565162951535312, 1.000000000000000000, 0.9510565162951535312, 1.000000000000000000, 0.9510565162951535312, 1.000000000000000000, 0.9510565162951535312, 1.000000000000000000, 0.9510565162951535312, 1.000000000000000000, 0.9510565162951535312, 1.000000000000000000, 0.9510565162951535312, 1.000000000000000000, 0.9510565162951535312, 1.000000000000000000, 0.9510565162951535312, 1.000000000000000000) ) ) 
 REPRESENTATION_ITEM ( '' )  SURFACE ( )  );
#24319=CARTESIAN_POINT ( 'NONE',  ( 15.00000000000000000, 73.35000000546237686, -4.873795443493596835 ) ) ;
#24352=FILL_AREA_STYLE ('',( #26915 ) ) ;
#24371=CYLINDRICAL_SURFACE ( 'NONE', #22631, 15.00000000000000000 ) ;
#24385=CARTESIAN_POINT ( 'NONE',  ( 2.688165632520823219E-15, 77.87500000273119838, 14.63369212191046387 ) ) ;
#24392=CARTESIAN_POINT ( 'NONE',  ( -8.601468415847515203, 75.67500000273116711, 11.83890561707634959 ) ) ;
#24396=ORIENTED_EDGE ( 'NONE', *, *, #20072, .T. ) ;
#24399=LINE ( 'NONE', #874, #11327 ) ;
#24407=CARTESIAN_POINT ( 'NONE',  ( 4.300734207923757602, 78.27500000273118985, -13.23629886949340673 ) ) ;
#24411=ORIENTED_EDGE ( 'NONE', *, *, #10090, .F. ) ;
#24445=LINE ( 'NONE', #8488, #22231 ) ;
#24474=EDGE_CURVE ( 'NONE', #22018, #23625, #2515, .T. ) ;
#24479=CARTESIAN_POINT ( 'NONE',  ( 4.300734207923761154, 77.47500000273116427, 13.23629886949340495 ) ) ;
#24532=CARTESIAN_POINT ( 'NONE',  ( 13.91746825000000065, 72.27500000273116143, 4.522059556121114987 ) ) ;
#24545=CARTESIAN_POINT ( 'NONE',  ( 8.601468415847520532, 74.07500000273121543, 11.83890561707634781 ) ) ;
#24554=CARTESIAN_POINT ( 'NONE',  ( -13.91746824999999887, 81.37500000273118417, 0.000000000000000000 ) ) ;
#24571=CARTESIAN_POINT ( 'NONE',  ( 11.25946833292375793, 78.07500000273121543, -8.180482586598735395 ) ) ;
#24575=ORIENTED_EDGE ( 'NONE', *, *, #19302, .F. ) ;
#24580=ORIENTED_EDGE ( 'NONE', *, *, #15609, .T. ) ;
#24608=CARTESIAN_POINT ( 'NONE',  ( -15.00000000000000000, 81.89999999999997726, -4.873795443493594171 ) ) ;
#24626=CARTESIAN_POINT ( 'NONE',  ( 12.13525491562421088, 75.05000000546240813, 8.816778784387095058 ) ) ;
#24639=CARTESIAN_POINT ( 'NONE',  ( 8.601468415847520532, 77.57500000273115859, 11.83890561707634781 ) ) ;
#24701=LINE ( 'NONE', #17163, #1470 ) ;
#24709=CARTESIAN_POINT ( 'NONE',  ( 15.00000000000000355, 80.90000000000000568, 4.873795443493592394 ) ) ;
#24720=CARTESIAN_POINT ( 'NONE',  ( -11.25946833292375793, 77.57500000273121543, 8.180482586598737171 ) ) ;
#24724=ORIENTED_EDGE ( 'NONE', *, *, #23732, .F. ) ;
#24735=CARTESIAN_POINT ( 'NONE',  ( -8.601468415847515203, 77.17500000273118133, 11.83890561707634959 ) ) ;
#24772=CARTESIAN_POINT ( 'NONE',  ( -13.91746824999999887, 80.87500000273118417, 0.000000000000000000 ) ) ;
#24790=CARTESIAN_POINT ( 'NONE',  ( -15.00000000000000000, 76.00000000000001421, 0.000000000000000000 ) ) ;
#24797=( BOUNDED_CURVE ( )  B_SPLINE_CURVE ( 2, ( #784, #26878, #22520, #5779, #17215, #16586, #3373, #27042, #24144, #29278, #11266, #19166, #612 ),
 .UNSPECIFIED., .F., .T. ) 
 B_SPLINE_CURVE_WITH_KNOTS ( ( 3, 2, 2, 2, 2, 2, 3 ),
 ( 0.2500000000000000000, 0.2600000000000000089, 0.2800000000000000266, 0.2999999999999999889, 0.3200000000000000067, 0.3400000000000000244, 0.3500000000000000333 ),
 .UNSPECIFIED. ) 
 CURVE ( )  GEOMETRIC_REPRESENTATION_ITEM ( )  RATIONAL_B_SPLINE_CURVE ( ( 0.9755282581475768211, 0.9755282581475768211, 1.000000000000000000, 0.9510565162951535312, 1.000000000000000000, 0.9510565162951535312, 1.000000000000000000, 0.9510565162951535312, 1.000000000000000000, 0.9510565162951535312, 1.000000000000000000, 0.9755282581475767101, 0.9755282581475768211 ) ) 
 REPRESENTATION_ITEM ( '' )  );
#24807=CARTESIAN_POINT ( 'NONE',  ( 8.601468415847516980, 74.17500000273122396, -11.83890561707634781 ) ) ;
#24818=CARTESIAN_POINT ( 'NONE',  ( -2.375766604868045029, 77.55125428154684641, -14.99999999999999822 ) ) ;
#24823=ORIENTED_EDGE ( 'NONE', *, *, #4738, .F. ) ;
#24837=CARTESIAN_POINT ( 'NONE',  ( 0.7848642672870491666, 74.00000000000002842, 14.13069591803647640 ) ) ;
#24876=CARTESIAN_POINT ( 'NONE',  ( -4.300734207923755825, 71.77500000273117564, 13.23629886949340673 ) ) ;
#24886=CARTESIAN_POINT ( 'NONE',  ( -8.960552108402744065E-16, 80.87500000273118417, -14.63369212191046209 ) ) ;
#24888=CARTESIAN_POINT ( 'NONE',  ( 2.897257156509938333E-15, 78.75000000546236834, 15.77193336357400710 ) ) ;
#24902=CARTESIAN_POINT ( 'NONE',  ( 13.91746825000000065, 71.77500000273117564, 4.522059556121114987 ) ) ;
#24943=VECTOR ( 'NONE', #9306, 1000.000000000000000 ) ;
#24955=CARTESIAN_POINT ( 'NONE',  ( -12.13525491562420910, 74.19999999999998863, 8.816778784387098611 ) ) ;
#24976=CARTESIAN_POINT ( 'NONE',  ( -11.25946833292375793, 74.67500000273119554, -8.180482586598733619 ) ) ;
#25017=CARTESIAN_POINT ( 'NONE',  ( -1.089172066684569321E-14, 76.75000000546238255, 15.00000000000000000 ) ) ;
#25037=ORIENTED_EDGE ( 'NONE', *, *, #2221, .F. ) ;
#25049=CARTESIAN_POINT ( 'NONE',  ( -4.635254915624208216, 80.39999999999997726, 14.26584774442730463 ) ) ;
#25057=CARTESIAN_POINT ( 'NONE',  ( 0.000000000000000000, 122.0000000000000000, -9.000000000000001776 ) ) ;
#25058=CARTESIAN_POINT ( 'NONE',  ( 4.300734207923757602, 76.77500000273118985, -13.23629886949340673 ) ) ;
#25060=CARTESIAN_POINT ( 'NONE',  ( 4.635254915624212657, 78.85000000546239107, 14.26584774442730286 ) ) ;
#25072=CARTESIAN_POINT ( 'NONE',  ( -8.601468415847515203, 73.17500000273119554, 11.83890561707634959 ) ) ;
#25120=VERTEX_POINT ( 'NONE', #25998 ) ;
#25125=ORIENTED_EDGE ( 'NONE', *, *, #18079, .T. ) ;
#25127=CARTESIAN_POINT ( 'NONE',  ( -2.375766604868041476, 74.44874571845313938, 14.99999999999999822 ) ) ;
#25128=ORIENTED_EDGE ( 'NONE', *, *, #1644, .T. ) ;
#25148=CARTESIAN_POINT ( 'NONE',  ( 11.25946833292375793, 76.07500000273120122, -8.180482586598735395 ) ) ;
#25166=ORIENTED_EDGE ( 'NONE', *, *, #4965, .F. ) ;
#25178=CARTESIAN_POINT ( 'NONE',  ( -7.755784534690364218, 74.00000000000002842, 12.20123439012139954 ) ) ;
#25199=CARTESIAN_POINT ( 'NONE',  ( -9.270509831248419985, 78.55000000546236549, 12.75976212528060039 ) ) ;
#25221=CARTESIAN_POINT ( 'NONE',  ( -11.25946833292375793, 73.57500000273120122, 8.180482586598737171 ) ) ;
#25235=CARTESIAN_POINT ( 'NONE',  ( 15.00000000000000355, 75.15000000546237402, 4.873795443493592394 ) ) ;
#25247=CARTESIAN_POINT ( 'NONE',  ( 8.601468415847520532, 80.07500000273120122, 11.83890561707634781 ) ) ;
#25278=ORIENTED_EDGE ( 'NONE', *, *, #32216, .T. ) ;
#25323=CARTESIAN_POINT ( 'NONE',  ( 8.601468415847520532, 71.57500000273118701, 11.83890561707634781 ) ) ;
#25351=CARTESIAN_POINT ( 'NONE',  ( 5.348221797398307942, 74.00000000000001421, 12.84883053416113974 ) ) ;
#25356=PRODUCT_CONTEXT ( 'NONE', #12045, 'mechanical' ) ;
#25377=EDGE_CURVE ( 'NONE', #4064, #11228, #29799, .T. ) ;
#25388=ORIENTED_EDGE ( 'NONE', *, *, #31175, .F. ) ;
#25393=CARTESIAN_POINT ( 'NONE',  ( 9.270509831248425314, 78.95000000546235697, 12.75976212528059683 ) ) ;
#25396=CARTESIAN_POINT ( 'NONE',  ( 15.00000000000000000, 79.10000000000000853, -4.873795443493596835 ) ) ;
#25407=CARTESIAN_POINT ( 'NONE',  ( -9.657523855033125146E-16, 75.75000000546241097, -15.77193336357400710 ) ) ;
#25414=CARTESIAN_POINT ( 'NONE',  ( -15.00000000000000000, 74.35000000546239107, 4.873795443493597723 ) ) ;
#25423=CARTESIAN_POINT ( 'NONE',  ( 8.601468415847516980, 72.17500000273116711, -11.83890561707634781 ) ) ;
#25430=ORIENTED_EDGE ( 'NONE', *, *, #32216, .F. ) ;
#25471=DIRECTION ( 'NONE',  ( 0.000000000000000000, -0.000000000000000000, -1.000000000000000000 ) ) ;
#25482=EDGE_LOOP ( 'NONE', ( #33312, #15787, #10880, #4402 ) ) ;
#25483=CARTESIAN_POINT ( 'NONE',  ( -4.635254915624208216, 76.40000000000001990, 14.26584774442730463 ) ) ;
#25493=PLANE ( 'NONE',  #31049 ) ;
#25521=CYLINDRICAL_SURFACE ( 'NONE', #19476, 12.00000000000000178 ) ;
#25529=CARTESIAN_POINT ( 'NONE',  ( 0.000000000000000000, 102.0000000000000284, -12.00000000000000178 ) ) ;
#25567=CARTESIAN_POINT ( 'NONE',  ( 8.891200544363830713E-16, 79.75000000546238255, -15.00000000000000000 ) ) ;
#25570=CARTESIAN_POINT ( 'NONE',  ( -4.635254915624208216, 76.40000000000001990, 14.26584774442730463 ) ) ;
#25577=EDGE_CURVE ( 'NONE', #22733, #4956, #11226, .T. ) ;
#25579=CARTESIAN_POINT ( 'NONE',  ( -11.25946833292375793, 75.17500000273119554, -8.180482586598733619 ) ) ;
#25581=CARTESIAN_POINT ( 'NONE',  ( 4.635254915624212657, 74.85000000546237686, 14.26584774442730286 ) ) ;
#25582=ORIENTED_EDGE ( 'NONE', *, *, #20645, .F. ) ;
#25595=CARTESIAN_POINT ( 'NONE',  ( 11.25946833292375793, 80.57500000273121543, -8.180482586598735395 ) ) ;
#25601=CARTESIAN_POINT ( 'NONE',  ( 9.270509831248425314, 78.70000000000001705, 12.75976212528059683 ) ) ;
#25727=CARTESIAN_POINT ( 'NONE',  ( 0.000000000000000000, 122.0000000000000000, 0.000000000000000000 ) ) ;
#25728=ORIENTED_EDGE ( 'NONE', *, *, #25377, .F. ) ;
#25736=CARTESIAN_POINT ( 'NONE',  ( 9.270509831248423538, 75.30000000000001137, -12.75976212528059861 ) ) ;
#25747=CARTESIAN_POINT ( 'NONE',  ( -12.13525491562420910, 72.45000000546237118, 8.816778784387098611 ) ) ;
#25752=CARTESIAN_POINT ( 'NONE',  ( -15.00000000000000000, 74.15000000546240244, -4.873795443493594171 ) ) ;
#25760=CARTESIAN_POINT ( 'NONE',  ( -8.601468415847515203, 77.67500000273122396, 11.83890561707634959 ) ) ;
#25805=FACE_OUTER_BOUND ( 'NONE', #893, .T. ) ;
#25809=DIRECTION ( 'NONE',  ( -0.000000000000000000, 1.000000000000000000, -0.000000000000000000 ) ) ;
#25853=DIRECTION ( 'NONE',  ( -0.000000000000000000, -1.000000000000000000, -0.000000000000000000 ) ) ;
#25867=SHAPE_DEFINITION_REPRESENTATION ( #15378, #3268 ) ;
#25880=PLANE ( 'NONE',  #10591 ) ;
#25891=VERTEX_POINT ( 'NONE', #8105 ) ;
#25896=ORIENTED_EDGE ( 'NONE', *, *, #15609, .F. ) ;
#25903=CARTESIAN_POINT ( 'NONE',  ( -15.00000000000000000, 75.89999999999996305, -4.873795443493594171 ) ) ;
#25921=VECTOR ( 'NONE', #333, 1000.000000000000000 ) ;
#25925=CARTESIAN_POINT ( 'NONE',  ( -13.91746824999999532, 74.77500000273120406, -4.522059556121115875 ) ) ;
#25928=CARTESIAN_POINT ( 'NONE',  ( 4.300734207923761154, 77.97500000273122112, 13.23629886949340495 ) ) ;
#25934=EDGE_CURVE ( 'NONE', #7233, #5684, #30338, .T. ) ;
#25998=CARTESIAN_POINT ( 'NONE',  ( 2.445080149700053643E-15, 74.50000000000000000, 15.00000000000000000 ) ) ;
#26013=CYLINDRICAL_SURFACE ( 'NONE', #8606, 9.000000000000001776 ) ;
#26027=ORIENTED_EDGE ( 'NONE', *, *, #33913, .F. ) ;
#26054=DIRECTION ( 'NONE',  ( 0.000000000000000000, 1.000000000000000000, 0.000000000000000000 ) ) ;
#26073=CARTESIAN_POINT ( 'NONE',  ( -11.54700538379251817, 96.00000000000002842, 19.99999999999999645 ) ) ;
#26077=CARTESIAN_POINT ( 'NONE',  ( 12.13525491562420910, 79.19999999999998863, -8.816778784387098611 ) ) ;
#26097=CARTESIAN_POINT ( 'NONE',  ( 11.25946833292375793, 74.07500000273120122, -8.180482586598735395 ) ) ;
#26100=CARTESIAN_POINT ( 'NONE',  ( -8.960552108402742093E-16, 78.87500000273118417, -14.63369212191046387 ) ) ;
#26133=AXIS2_PLACEMENT_3D ( 'NONE', #14437, #27475, #21665 ) ;
#26150=CARTESIAN_POINT ( 'NONE',  ( -23.09401076758502924, 96.00000000000002842, 5.354274672883389237E-15 ) ) ;
#26156=EDGE_LOOP ( 'NONE', ( #22984, #33182, #27512, #8627 ) ) ;
#26240=EDGE_CURVE ( 'NONE', #28702, #220, #13432, .T. ) ;
#26258=CARTESIAN_POINT ( 'NONE',  ( 9.724104179731403619, 74.00000000000002842, -10.28132335189565083 ) ) ;
#26267=DIRECTION ( 'NONE',  ( -0.000000000000000000, -1.000000000000000000, -0.000000000000000000 ) ) ;
#26268=CARTESIAN_POINT ( 'NONE',  ( 8.601468415847520532, 75.57500000273117280, 11.83890561707634603 ) ) ;
#26271=CARTESIAN_POINT ( 'NONE',  ( -4.300734207923755825, 79.77500000273118985, 13.23629886949340673 ) ) ;
#26279=EDGE_LOOP ( 'NONE', ( #19310, #19987, #7769, #11695 ) ) ;
#26292=CARTESIAN_POINT ( 'NONE',  ( 13.21205807576171232, 74.00000000000002842, -4.468464182411219454 ) ) ;
#26366=DIRECTION ( 'NONE',  ( -0.000000000000000000, 1.000000000000000000, -0.000000000000000000 ) ) ;
#26389=CARTESIAN_POINT ( 'NONE',  ( -15.00000000000000000, 72.25000000546238255, 0.000000000000000000 ) ) ;
#26404=CONICAL_SURFACE ( 'NONE', #6640, 14.00000000000000178, 0.2617993877991500740 ) ;
#26438=CARTESIAN_POINT ( 'NONE',  ( 13.91746824999999887, 77.87500000273116996, -1.704398294459741270E-15 ) ) ;
#26441=CARTESIAN_POINT ( 'NONE',  ( -13.91746824999999532, 79.27500000273117564, -4.522059556121115875 ) ) ;
#26443=AXIS2_PLACEMENT_3D ( 'NONE', #921, #6078, #32162 ) ;
#26456=CARTESIAN_POINT ( 'NONE',  ( 11.25946833292375793, 76.57500000273120122, -8.180482586598735395 ) ) ;
#26458=CARTESIAN_POINT ( 'NONE',  ( -15.00000000000000000, 76.15000000546238823, -4.873795443493594171 ) ) ;
#26460=CARTESIAN_POINT ( 'NONE',  ( 13.91805153345283230, 74.00000000000007105, -0.9002929780893395018 ) ) ;
#26490=CARTESIAN_POINT ( 'NONE',  ( 15.00000000000000000, 77.00000000000001421, -1.836970198721029589E-15 ) ) ;
#26497=VERTEX_POINT ( 'NONE', #21493 ) ;
#26531=CARTESIAN_POINT ( 'NONE',  ( 8.891200544363830713E-16, 81.50000000000000000, -15.00000000000000000 ) ) ;
#26557=CARTESIAN_POINT ( 'NONE',  ( 4.635254915624209993, 71.65000000546240244, -14.26584774442730463 ) ) ;
#26560=LINE ( 'NONE', #13527, #17167 ) ;
#26573=ADVANCED_FACE ( 'NONE', ( #868 ), #31025, .T. ) ;
#26576=EDGE_CURVE ( 'NONE', #20845, #25120, #20522, .T. ) ;
#26595=CARTESIAN_POINT ( 'NONE',  ( -5.580114035484361246, 74.00000000000002842, -13.73609794928142058 ) ) ;
#26606=CARTESIAN_POINT ( 'NONE',  ( -11.25946833292375793, 75.07500000273120122, 8.180482586598737171 ) ) ;
#26609=AXIS2_PLACEMENT_3D ( 'NONE', #3123, #31433, #31931 ) ;
#26610=CARTESIAN_POINT ( 'NONE',  ( -13.91746824999999887, 73.37500000273116996, 0.000000000000000000 ) ) ;
#26616=VERTEX_POINT ( 'NONE', #28238 ) ;
#26625=CARTESIAN_POINT ( 'NONE',  ( 4.300734207923761154, 77.97500000273122112, 13.23629886949340495 ) ) ;
#26629=FACE_OUTER_BOUND ( 'NONE', #8807, .T. ) ;
#26643=CIRCLE ( 'NONE', #28838, 11.32050807568876749 ) ;
#26669=EDGE_CURVE ( 'NONE', #17411, #19608, #16803, .T. ) ;
#26704=FACE_BOUND ( 'NONE', #5472, .T. ) ;
#26707=CARTESIAN_POINT ( 'NONE',  ( -11.54700538379251817, 96.00000000000002842, 19.99999999999999645 ) ) ;
#26725=CARTESIAN_POINT ( 'NONE',  ( -13.91746824999999532, 78.97500000273117848, 4.522059556121122093 ) ) ;
#26733=DIRECTION ( 'NONE',  ( -0.000000000000000000, -1.000000000000000000, -0.000000000000000000 ) ) ;
#26752=CARTESIAN_POINT ( 'NONE',  ( -9.657523855033125146E-16, 73.50000000000001421, -15.77193336357400710 ) ) ;
#26756=SURFACE_SIDE_STYLE ('',( #29987 ) ) ;
#26773=LINE ( 'NONE', #3263, #13901 ) ;
#26790=CARTESIAN_POINT ( 'NONE',  ( 13.91746824999999887, 80.37500000273118417, -1.704398294459741270E-15 ) ) ;
#26794=CARTESIAN_POINT ( 'NONE',  ( 13.82681134000903356, 73.99999999999998579, 1.827769615135852233 ) ) ;
#26815=CARTESIAN_POINT ( 'NONE',  ( 13.91746824999999532, 75.97500000273116427, -4.522059556121118540 ) ) ;
#26825=ORIENTED_EDGE ( 'NONE', *, *, #7949, .F. ) ;
#26841=ORIENTED_EDGE ( 'NONE', *, *, #18514, .F. ) ;
#26878=CARTESIAN_POINT ( 'NONE',  ( 2.375766604868043252, 77.69874572391549350, -14.99999999999999822 ) ) ;
#26886=CARTESIAN_POINT ( 'NONE',  ( -11.25946833292375793, 78.67500000273119554, -8.180482586598733619 ) ) ;
#26891=CARTESIAN_POINT ( 'NONE',  ( -9.270509831248419985, 80.30000000000002558, 12.75976212528060039 ) ) ;
#26895=CYLINDRICAL_SURFACE ( 'NONE', #2881, 15.00000000000000000 ) ;
#26915=FILL_AREA_STYLE_COLOUR ( '', #12287 ) ;
#26948=CARTESIAN_POINT ( 'NONE',  ( -13.91746824999999532, 79.27500000273117564, -4.522059556121115875 ) ) ;
#26961=ORIENTED_EDGE ( 'NONE', *, *, #18507, .F. ) ;
#26972=ADVANCED_FACE ( 'NONE', ( #17422 ), #33184, .F. ) ;
#26973=CARTESIAN_POINT ( 'NONE',  ( -4.300734207923759378, 76.47500000273116427, -13.23629886949340495 ) ) ;
#27042=CARTESIAN_POINT ( 'NONE',  ( 15.00000000000000355, 77.15000000546235981, 4.873795443493592394 ) ) ;
#27051=CARTESIAN_POINT ( 'NONE',  ( -11.25946833292375793, 77.07500000273121543, 8.180482586598737171 ) ) ;
#27056=CARTESIAN_POINT ( 'NONE',  ( -4.635254915624211769, 79.85000000546239107, -14.26584774442730286 ) ) ;
#27079=EDGE_CURVE ( 'NONE', #22980, #20845, #6267, .T. ) ;
#27097=CARTESIAN_POINT ( 'NONE',  ( -11.54700538379251995, 96.00000000000002842, -19.99999999999999645 ) ) ;
#27105=CARTESIAN_POINT ( 'NONE',  ( 11.25946833292375793, 72.57500000273120122, -8.180482586598735395 ) ) ;
#27121=CARTESIAN_POINT ( 'NONE',  ( 15.00000000000000000, 81.09999999999999432, -4.873795443493596835 ) ) ;
#27158=ORIENTED_EDGE ( 'NONE', *, *, #21264, .F. ) ;
#27201=DIRECTION ( 'NONE',  ( 0.000000000000000000, 1.000000000000000000, 0.000000000000000000 ) ) ;
#27212=DIRECTION ( 'NONE',  ( 0.000000000000000000, 0.000000000000000000, 1.000000000000000000 ) ) ;
#27220=CARTESIAN_POINT ( 'NONE',  ( -13.91746824999999532, 72.77500000273120406, -4.522059556121115875 ) ) ;
#27224=CARTESIAN_POINT ( 'NONE',  ( 0.000000000000000000, 102.0000000000000284, 0.000000000000000000 ) ) ;
#27244=DIRECTION ( 'NONE',  ( -0.000000000000000000, 1.000000000000000000, -0.000000000000000000 ) ) ;
#27289=CARTESIAN_POINT ( 'NONE',  ( -15.00000000000000000, 82.00000000000001421, 0.000000000000000000 ) ) ;
#27299=CARTESIAN_POINT ( 'NONE',  ( -11.25946833292375793, 79.17500000273119554, -8.180482586598733619 ) ) ;
#27316=CARTESIAN_POINT ( 'NONE',  ( 2.688165632520823219E-15, 77.37500000273118417, 14.63369212191046387 ) ) ;
#27327=EDGE_LOOP ( 'NONE', ( #14282, #30093, #21704, #29926 ) ) ;
#27340=CARTESIAN_POINT ( 'NONE',  ( 11.54700538379251107, 96.00000000000002842, -19.99999999999999645 ) ) ;
#27348=PLANE ( 'NONE',  #13242 ) ;
#27357=CARTESIAN_POINT ( 'NONE',  ( 8.891200544363830713E-16, 81.50000000000001421, -15.00000000000000000 ) ) ;
#27360=FILL_AREA_STYLE_COLOUR ( '', #818 ) ;
#27370=DIRECTION ( 'NONE',  ( 0.5000000000000000000, 0.000000000000000000, 0.8660254037844385966 ) ) ;
#27388=CARTESIAN_POINT ( 'NONE',  ( 13.91746824999999887, 73.87500000273116996, -1.704398294459741270E-15 ) ) ;
#27405=ORIENTED_EDGE ( 'NONE', *, *, #7993, .T. ) ;
#27456=CARTESIAN_POINT ( 'NONE',  ( -4.300734207923755825, 73.77500000273118985, 13.23629886949340673 ) ) ;
#27460=DIRECTION ( 'NONE',  ( 0.000000000000000000, 0.000000000000000000, 1.000000000000000000 ) ) ;
#27468=CARTESIAN_POINT ( 'NONE',  ( 13.91746825000000065, 76.27500000273116143, 4.522059556121115875 ) ) ;
#27475=DIRECTION ( 'NONE',  ( -0.000000000000000000, 1.000000000000000000, -0.000000000000000000 ) ) ;
#27483=CARTESIAN_POINT ( 'NONE',  ( -8.960552108402742093E-16, 80.37500000273118417, -14.63369212191046387 ) ) ;
#27490=AXIS2_PLACEMENT_3D ( 'NONE', #31180, #2701, #2352 ) ;
#27503=EDGE_CURVE ( 'NONE', #3774, #15262, #731, .T. ) ;
#27509=DIRECTION ( 'NONE',  ( 0.000000000000000000, 0.000000000000000000, 1.000000000000000000 ) ) ;
#27512=ORIENTED_EDGE ( 'NONE', *, *, #17994, .T. ) ;
#27514=DIRECTION ( 'NONE',  ( 0.5000000000000002220, 0.000000000000000000, 0.8660254037844384856 ) ) ;
#27527=ORIENTED_EDGE ( 'NONE', *, *, #25377, .T. ) ;
#27555=CARTESIAN_POINT ( 'NONE',  ( 13.91746825000000065, 75.77500000273117564, 4.522059556121114987 ) ) ;
#27562=CARTESIAN_POINT ( 'NONE',  ( 0.000000000000000000, 74.00000000000001421, 15.00000000000000000 ) ) ;
#27575=ORIENTED_EDGE ( 'NONE', *, *, #28553, .T. ) ;
#27620=DIRECTION ( 'NONE',  ( -0.000000000000000000, 1.000000000000000000, -0.000000000000000000 ) ) ;
#27628=CARTESIAN_POINT ( 'NONE',  ( 2.688165632520823219E-15, 71.87500000273116996, 14.63369212191046387 ) ) ;
#27631=VECTOR ( 'NONE', #23412, 1000.000000000000227 ) ;
#27638=CARTESIAN_POINT ( 'NONE',  ( -8.960552108402744065E-16, 78.87500000273118417, -14.63369212191046209 ) ) ;
#27640=CARTESIAN_POINT ( 'NONE',  ( -12.13525491562420910, 74.45000000546237118, 8.816778784387098611 ) ) ;
#27645=CARTESIAN_POINT ( 'NONE',  ( -2.375766604868041476, 74.69874572391553613, 14.99999999999999822 ) ) ;
#27653=CARTESIAN_POINT ( 'NONE',  ( 11.25946833292375793, 75.67500000273119554, 8.180482586598731842 ) ) ;
#27660=EDGE_LOOP ( 'NONE', ( #25166, #3794 ) ) ;
#27672=MECHANICAL_DESIGN_GEOMETRIC_PRESENTATION_REPRESENTATION('',(#18367),#7940);
#27697=CONICAL_SURFACE ( 'NONE', #26609, 13.32050807568876927, 0.2617993877991500740 ) ;
#27704=ORIENTED_EDGE ( 'NONE', *, *, #12358, .T. ) ;
#27713=( BOUNDED_CURVE ( )  B_SPLINE_CURVE ( 2, ( #7402, #7055, #9632, #17199, #20457, #30908, #33309, #30384, #14961, #25601, #12032, #17888, #15137 ),
 .UNSPECIFIED., .F., .T. ) 
 B_SPLINE_CURVE_WITH_KNOTS ( ( 3, 2, 2, 2, 2, 2, 3 ),
 ( 0.2500000000000000000, 0.2600000000000000089, 0.2800000000000000266, 0.2999999999999999889, 0.3200000000000000067, 0.3400000000000000244, 0.3500000000000000333 ),
 .UNSPECIFIED. ) 
 CURVE ( )  GEOMETRIC_REPRESENTATION_ITEM ( )  RATIONAL_B_SPLINE_CURVE ( ( 0.9755282581475768211, 0.9755282581475768211, 1.000000000000000000, 0.9510565162951535312, 1.000000000000000000, 0.9510565162951535312, 1.000000000000000000, 0.9510565162951535312, 1.000000000000000000, 0.9510565162951535312, 1.000000000000000000, 0.9755282581475767101, 0.9755282581475768211 ) ) 
 REPRESENTATION_ITEM ( '' )  );
#27727=CARTESIAN_POINT ( 'NONE',  ( -13.91746824999999887, 72.87500000273122680, 0.000000000000000000 ) ) ;
#27800=CARTESIAN_POINT ( 'NONE',  ( 13.91746825000000065, 74.27500000273120406, 4.522059556121114987 ) ) ;
#27809=CARTESIAN_POINT ( 'NONE',  ( 2.688165632520823219E-15, 75.87500000273115575, 14.63369212191046209 ) ) ;
#27811=CARTESIAN_POINT ( 'NONE',  ( 4.635254915624212657, 76.85000000546237686, 14.26584774442730286 ) ) ;
#27825=CARTESIAN_POINT ( 'NONE',  ( 11.25946833292375793, 71.67500000273119554, 8.180482586598731842 ) ) ;
#27838=ORIENTED_EDGE ( 'NONE', *, *, #29363, .F. ) ;
#27847=AXIS2_PLACEMENT_3D ( 'NONE', #17827, #12843, #10609 ) ;
#27849=CARTESIAN_POINT ( 'NONE',  ( -8.891200544363830713E-16, 79.49999999999998579, -15.00000000000000000 ) ) ;
#27859=CARTESIAN_POINT ( 'NONE',  ( 0.000000000000000000, 74.00000000000001421, 15.00000000000000000 ) ) ;
#27881=ORIENTED_EDGE ( 'NONE', *, *, #29583, .T. ) ;
#27910=CARTESIAN_POINT ( 'NONE',  ( -15.00000000000000000, 78.09999999999998010, 4.873795443493597723 ) ) ;
#27970=CARTESIAN_POINT ( 'NONE',  ( -12.13525491562421088, 73.80000000000002558, -8.816778784387096835 ) ) ;
#27979=CARTESIAN_POINT ( 'NONE',  ( 13.91746824999999887, 74.37500000273116996, -1.704398294459741270E-15 ) ) ;
#27981=CARTESIAN_POINT ( 'NONE',  ( 9.270509831248425314, 78.95000000546235697, 12.75976212528059683 ) ) ;
#27994=CARTESIAN_POINT ( 'NONE',  ( 8.601468415847520532, 73.57500000273117280, 11.83890561707634781 ) ) ;
#28072=CARTESIAN_POINT ( 'NONE',  ( -8.891200544363830713E-16, 75.75000000546238255, -15.00000000000000000 ) ) ;
#28076=CARTESIAN_POINT ( 'NONE',  ( -15.00000000000000000, 78.00000000000001421, 0.000000000000000000 ) ) ;
#28098=CARTESIAN_POINT ( 'NONE',  ( -7.239203213863182995, 74.00000000000001421, 12.48853769527896951 ) ) ;
#28140=CARTESIAN_POINT ( 'NONE',  ( -15.00000000000000000, 78.00000000000001421, 0.000000000000000000 ) ) ;
#28152=CARTESIAN_POINT ( 'NONE',  ( -15.00000000000000000, 76.25000000546239676, 0.000000000000000000 ) ) ;
#28165=CARTESIAN_POINT ( 'NONE',  ( 2.688165632520823219E-15, 73.37500000273118417, 14.63369212191046387 ) ) ;
#28226=DIRECTION ( 'NONE',  ( -0.000000000000000000, -1.000000000000000000, -0.000000000000000000 ) ) ;
#28231=DIRECTION ( 'NONE',  ( -0.000000000000000000, -1.000000000000000000, -0.000000000000000000 ) ) ;
#28238=CARTESIAN_POINT ( 'NONE',  ( -15.00000000000000000, 82.00000000000001421, 0.000000000000000000 ) ) ;
#28299=DIRECTION ( 'NONE',  ( 0.000000000000000000, 0.000000000000000000, 1.000000000000000000 ) ) ;
#28308=CARTESIAN_POINT ( 'NONE',  ( 15.00000000000000000, 75.00000000000001421, -1.836970198721029589E-15 ) ) ;
#28320=CARTESIAN_POINT ( 'NONE',  ( -12.13525491562420910, 70.45000000546237118, 8.816778784387098611 ) ) ;
#28324=ADVANCED_FACE ( 'NONE', ( #6018 ), #31918, .T. ) ;
#28327=CARTESIAN_POINT ( 'NONE',  ( 11.54700538379251107, 86.00000000000001421, -19.99999999999999645 ) ) ;
#28335=CARTESIAN_POINT ( 'NONE',  ( -8.960552108402742093E-16, 76.87500000273118417, -14.63369212191046387 ) ) ;
#28344=ORIENTED_EDGE ( 'NONE', *, *, #18507, .T. ) ;
#28408=CARTESIAN_POINT ( 'NONE',  ( 12.13525491562421088, 74.80000000000003979, 8.816778784387095058 ) ) ;
#28436=CARTESIAN_POINT ( 'NONE',  ( 0.000000000000000000, 96.00000000000002842, -12.00000000000000000 ) ) ;
#28475=CARTESIAN_POINT ( 'NONE',  ( 15.00000000000000000, 77.00000000000001421, -1.836970198721029589E-15 ) ) ;
#28496=CARTESIAN_POINT ( 'NONE',  ( 4.300734207923757602, 76.77500000273118985, -13.23629886949340673 ) ) ;
#28497=CARTESIAN_POINT ( 'NONE',  ( -13.91746824999999532, 78.77500000273118985, -4.522059556121115875 ) ) ;
#28543=FACE_BOUND ( 'NONE', #30199, .T. ) ;
#28553=EDGE_CURVE ( 'NONE', #19151, #5214, #15533, .T. ) ;
#28564=CARTESIAN_POINT ( 'NONE',  ( 12.13525491562421088, 80.79999999999998295, 8.816778784387095058 ) ) ;
#28632=ORIENTED_EDGE ( 'NONE', *, *, #16303, .T. ) ;
#28642=CARTESIAN_POINT ( 'NONE',  ( 9.270509831248425314, 74.69999999999994600, 12.75976212528059683 ) ) ;
#28656=EDGE_CURVE ( 'NONE', #871, #220, #33540, .T. ) ;
#28668=CARTESIAN_POINT ( 'NONE',  ( 2.688165632520823219E-15, 77.37500000273116996, 14.63369212191046209 ) ) ;
#28671=CARTESIAN_POINT ( 'NONE',  ( -13.91746824999999532, 79.47500000273115006, 4.522059556121122093 ) ) ;
#28673=LINE ( 'NONE', #12722, #32395 ) ;
#28702=VERTEX_POINT ( 'NONE', #23387 ) ;
#28737=CARTESIAN_POINT ( 'NONE',  ( -4.223320258572821363E-15, 80.50000000000001421, 15.00000000000000355 ) ) ;
#28767=CARTESIAN_POINT ( 'NONE',  ( 0.000000000000000000, 102.0000000000000284, -12.00000000000000178 ) ) ;
#28806=VERTEX_POINT ( 'NONE', #23263 ) ;
#28814=CARTESIAN_POINT ( 'NONE',  ( 9.270509831248425314, 72.70000000000004547, 12.75976212528059683 ) ) ;
#28834=CARTESIAN_POINT ( 'NONE',  ( -8.601468415847515203, 77.17500000273118133, 11.83890561707634959 ) ) ;
#28837=CARTESIAN_POINT ( 'NONE',  ( 11.25946833292375793, 78.57500000273121543, -8.180482586598735395 ) ) ;
#28838=AXIS2_PLACEMENT_3D ( 'NONE', #21496, #16019, #16187 ) ;
#28858=EDGE_CURVE ( 'NONE', #5592, #8282, #19017, .T. ) ;
#28866=CARTESIAN_POINT ( 'NONE',  ( -1.714505518806294835E-15, 102.0000000000000284, -14.00000000000000178 ) ) ;
#28890=ORIENTED_EDGE ( 'NONE', *, *, #26576, .F. ) ;
#28929=ORIENTED_EDGE ( 'NONE', *, *, #23684, .T. ) ;
#28931=DIRECTION ( 'NONE',  ( 0.000000000000000000, 0.000000000000000000, 1.000000000000000000 ) ) ;
#28956=CARTESIAN_POINT ( 'NONE',  ( -8.960552108402742093E-16, 78.37500000273119838, -14.63369212191046387 ) ) ;
#28982=ADVANCED_FACE ( 'NONE', ( #12959 ), #31941, .T. ) ;
#28983=CARTESIAN_POINT ( 'NONE',  ( 2.897257156509938333E-15, 72.50000000000004263, 15.77193336357400710 ) ) ;
#29001=CARTESIAN_POINT ( 'NONE',  ( -11.25946833292375793, 78.67500000273119554, -8.180482586598733619 ) ) ;
#29004=CARTESIAN_POINT ( 'NONE',  ( -11.25946833292375793, 77.17500000273119554, -8.180482586598733619 ) ) ;
#29019=CARTESIAN_POINT ( 'NONE',  ( -13.91746824999999887, 77.37500000273116996, 0.000000000000000000 ) ) ;
#29021=CARTESIAN_POINT ( 'NONE',  ( -15.00000000000000000, 76.35000000546239107, 4.873795443493597723 ) ) ;
#29088=ORIENTED_EDGE ( 'NONE', *, *, #22904, .T. ) ;
#29119=CARTESIAN_POINT ( 'NONE',  ( 2.897257156509938333E-15, 72.75000000546239676, 15.77193336357400710 ) ) ;
#29162=ADVANCED_BREP_SHAPE_REPRESENTATION ( '', ( #32070, #1376 ), #19430 ) ;
#29165=CARTESIAN_POINT ( 'NONE',  ( 8.601468415847516980, 80.17500000273112448, -11.83890561707634603 ) ) ;
#29169=CARTESIAN_POINT ( 'NONE',  ( -13.91746824999999532, 73.47500000273117848, 4.522059556121122093 ) ) ;
#29186=CARTESIAN_POINT ( 'NONE',  ( -11.25946833292375793, 77.57500000273121543, 8.180482586598737171 ) ) ;
#29188=CARTESIAN_POINT ( 'NONE',  ( -2.375766604868045029, 75.80125428700922896, -14.99999999999999822 ) ) ;
#29190=CARTESIAN_POINT ( 'NONE',  ( 12.51014164588334232, 74.00000000000002842, 6.166118349127116538 ) ) ;
#29197=CARTESIAN_POINT ( 'NONE',  ( 0.000000000000000000, 111.9999999999999858, 13.32050807568876927 ) ) ;
#29220=CARTESIAN_POINT ( 'NONE',  ( 9.270509831248421762, 77.30000000000001137, -12.75976212528059861 ) ) ;
#29225=CIRCLE ( 'NONE', #14410, 11.32050807568876749 ) ;
#29234=EDGE_CURVE ( 'NONE', #4172, #12253, #10515, .T. ) ;
#29278=CARTESIAN_POINT ( 'NONE',  ( 9.270509831248425314, 76.95000000546237118, 12.75976212528059683 ) ) ;
#29283=DIRECTION ( 'NONE',  ( 0.000000000000000000, 0.000000000000000000, 1.000000000000000000 ) ) ;
#29287=CARTESIAN_POINT ( 'NONE',  ( -15.00000000000000000, 70.35000000546234844, 4.873795443493597723 ) ) ;
#29325=CARTESIAN_POINT ( 'NONE',  ( 7.965081083986921939, 73.99999999999998579, -11.86478431723531912 ) ) ;
#29355=CARTESIAN_POINT ( 'NONE',  ( -4.300734207923759378, 80.97500000273122112, -13.23629886949340495 ) ) ;
#29363=EDGE_CURVE ( 'NONE', #16782, #26497, #33004, .T. ) ;
#29409=ORIENTED_EDGE ( 'NONE', *, *, #4947, .T. ) ;
#29437=CARTESIAN_POINT ( 'NONE',  ( 4.635254915624212657, 74.85000000546237686, 14.26584774442730286 ) ) ;
#29452=CARTESIAN_POINT ( 'NONE',  ( 13.91746825000000065, 79.77500000273116143, 4.522059556121114987 ) ) ;
#29511=LINE ( 'NONE', #10838, #3690 ) ;
#29514=CARTESIAN_POINT ( 'NONE',  ( 8.601468415847520532, 78.07500000273120122, 11.83890561707634781 ) ) ;
#29522=DIRECTION ( 'NONE',  ( 0.000000000000000000, 0.000000000000000000, -1.000000000000000000 ) ) ;
#29538=FACE_OUTER_BOUND ( 'NONE', #10753, .T. ) ;
#29583=EDGE_CURVE ( 'NONE', #17758, #16375, #6, .T. ) ;
#29584=ORIENTED_EDGE ( 'NONE', *, *, #25577, .F. ) ;
#29611=CARTESIAN_POINT ( 'NONE',  ( 13.91746824999999532, 71.97500000273117848, -4.522059556121118540 ) ) ;
#29621=CARTESIAN_POINT ( 'NONE',  ( 0.000000000000000000, 74.00000000000001421, 0.000000000000000000 ) ) ;
#29663=CARTESIAN_POINT ( 'NONE',  ( -13.91746824999999532, 71.47500000273119269, 4.522059556121122093 ) ) ;
#29677=CARTESIAN_POINT ( 'NONE',  ( -8.601468415847515203, 77.67500000273122396, 11.83890561707634959 ) ) ;
#29686=CARTESIAN_POINT ( 'NONE',  ( -13.91746824999999887, 77.37500000273116996, 0.000000000000000000 ) ) ;
#29689=ADVANCED_FACE ( 'NONE', ( #20209 ), #15398, .T. ) ;
#29704=CARTESIAN_POINT ( 'NONE',  ( 11.25946833292375793, 79.67500000273119554, 8.180482586598731842 ) ) ;
#29760=VERTEX_POINT ( 'NONE', #17802 ) ;
#29780=CARTESIAN_POINT ( 'NONE',  ( 13.91746825000000065, 77.77500000273114722, 4.522059556121114987 ) ) ;
#29786=DIRECTION ( 'NONE',  ( 0.000000000000000000, 0.000000000000000000, 1.000000000000000000 ) ) ;
#29787=CARTESIAN_POINT ( 'NONE',  ( -12.13525491562420910, 80.19999999999998863, 8.816778784387098611 ) ) ;
#29799=CIRCLE ( 'NONE', #754, 9.000000000000001776 ) ;
#29803=( BOUNDED_CURVE ( )  B_SPLINE_CURVE ( 2, ( #14189, #31865, #8860, #26891, #29787, #3550, #11439, #18847, #14022, #22086, #32033, #21759, #21916 ),
 .UNSPECIFIED., .F., .T. ) 
 B_SPLINE_CURVE_WITH_KNOTS ( ( 3, 2, 2, 2, 2, 2, 3 ),
 ( 0.1500000000000000222, 0.1600000000000000033, 0.1799999999999999933, 0.2000000000000000111, 0.2200000000000000011, 0.2399999999999999911, 0.2500000000000000000 ),
 .UNSPECIFIED. ) 
 CURVE ( )  GEOMETRIC_REPRESENTATION_ITEM ( )  RATIONAL_B_SPLINE_CURVE ( ( 0.9755282581475768211, 0.9755282581475768211, 1.000000000000000000, 0.9510565162951535312, 1.000000000000000000, 0.9510565162951535312, 1.000000000000000000, 0.9510565162951535312, 1.000000000000000000, 0.9510565162951535312, 1.000000000000000000, 0.9755282581475768211, 0.9755282581475768211 ) ) 
 REPRESENTATION_ITEM ( '' )  );
#29820=( GEOMETRIC_REPRESENTATION_CONTEXT ( 3 ) GLOBAL_UNCERTAINTY_ASSIGNED_CONTEXT ( ( #11645 ) ) GLOBAL_UNIT_ASSIGNED_CONTEXT ( ( #8558, #11803, #32724 ) ) REPRESENTATION_CONTEXT ( 'NONE', 'WORKASPACE' ) );
#29854=CARTESIAN_POINT ( 'NONE',  ( -9.657523855033125146E-16, 81.50000000000000000, -15.77193336357400710 ) ) ;
#29864=CARTESIAN_POINT ( 'NONE',  ( 11.25946833292375793, 78.17500000273119554, 8.180482586598731842 ) ) ;
#29868=ORIENTED_EDGE ( 'NONE', *, *, #7432, .F. ) ;
#29880=CARTESIAN_POINT ( 'NONE',  ( 13.91746824999999532, 77.97500000273122112, -4.522059556121118540 ) ) ;
#29884=ORIENTED_EDGE ( 'NONE', *, *, #30099, .F. ) ;
#29890=VERTEX_POINT ( 'NONE', #28767 ) ;
#29910=DIRECTION ( 'NONE',  ( 0.4999999999999997224, 0.000000000000000000, -0.8660254037844387076 ) ) ;
#29912=EDGE_CURVE ( 'NONE', #9084, #4172, #29225, .T. ) ;
#29926=ORIENTED_EDGE ( 'NONE', *, *, #17205, .F. ) ;
#29952=CARTESIAN_POINT ( 'NONE',  ( -8.960552108402742093E-16, 74.37500000273121259, -14.63369212191046387 ) ) ;
#29982=FACE_OUTER_BOUND ( 'NONE', #25482, .T. ) ;
#29987=SURFACE_STYLE_FILL_AREA ( #24352 ) ;
#29999=FACE_OUTER_BOUND ( 'NONE', #33532, .T. ) ;
#30022=CARTESIAN_POINT ( 'NONE',  ( -9.270509831248421762, 80.30000000000002558, 12.75976212528060039 ) ) ;
#30031=CARTESIAN_POINT ( 'NONE',  ( 13.91746824999999532, 80.47500000273119269, -4.522059556121118540 ) ) ;
#30037=CARTESIAN_POINT ( 'NONE',  ( 0.000000000000000000, 102.0000000000000284, 0.000000000000000000 ) ) ;
#30045=CARTESIAN_POINT ( 'NONE',  ( -13.91746824999999532, 76.97500000273119269, 4.522059556121122093 ) ) ;
#30053=VERTEX_POINT ( 'NONE', #26707 ) ;
#30055=EDGE_LOOP ( 'NONE', ( #8783, #11389 ) ) ;
#30093=ORIENTED_EDGE ( 'NONE', *, *, #30099, .T. ) ;
#30099=EDGE_CURVE ( 'NONE', #4064, #5214, #5433, .T. ) ;
#30109=FACE_BOUND ( 'NONE', #15531, .T. ) ;
#30114=CARTESIAN_POINT ( 'NONE',  ( 8.601468415847516980, 72.17500000273116711, -11.83890561707634781 ) ) ;
#30121=LINE ( 'NONE', #27562, #31071 ) ;
#30164=CARTESIAN_POINT ( 'NONE',  ( -15.00000000000000000, 81.12500000273121259, 0.000000000000000000 ) ) ;
#30171=VECTOR ( 'NONE', #14549, 1000.000000000000000 ) ;
#30184=CARTESIAN_POINT ( 'NONE',  ( -4.300734207923759378, 72.97500000273122112, -13.23629886949340495 ) ) ;
#30195=AXIS2_PLACEMENT_3D ( 'NONE', #22639, #26366, #28931 ) ;
#30196=CARTESIAN_POINT ( 'NONE',  ( -4.300734207923755825, 77.77500000273118985, 13.23629886949340673 ) ) ;
#30198=CARTESIAN_POINT ( 'NONE',  ( -4.635254915624211769, 75.85000000546237686, -14.26584774442730286 ) ) ;
#30199=EDGE_LOOP ( 'NONE', ( #30956, #31508 ) ) ;
#30209=ADVANCED_FACE ( 'NONE', ( #23696 ), #5331, .F. ) ;
#30212=CARTESIAN_POINT ( 'NONE',  ( 13.91746825000000065, 80.27500000273120406, 4.522059556121114987 ) ) ;
#30216=ORIENTED_EDGE ( 'NONE', *, *, #20645, .T. ) ;
#30219=VECTOR ( 'NONE', #23468, 1000.000000000000000 ) ;
#30239=CARTESIAN_POINT ( 'NONE',  ( 11.54700538379251107, 86.00000000000001421, -19.99999999999999645 ) ) ;
#30246=EDGE_CURVE ( 'NONE', #5684, #7233, #8401, .T. ) ;
#30254=ORIENTED_EDGE ( 'NONE', *, *, #9790, .T. ) ;
#30285=CARTESIAN_POINT ( 'NONE',  ( -4.300734207923755825, 77.27500000273118985, 13.23629886949340673 ) ) ;
#30294=CARTESIAN_POINT ( 'NONE',  ( -8.891200544363830713E-16, 77.49999999999998579, -15.00000000000000000 ) ) ;
#30301=ORIENTED_EDGE ( 'NONE', *, *, #18121, .T. ) ;
#30338=CIRCLE ( 'NONE', #13923, 15.00000000000000000 ) ;
#30356=CARTESIAN_POINT ( 'NONE',  ( 11.25946833292375793, 74.57500000273120122, -8.180482586598735395 ) ) ;
#30366=CARTESIAN_POINT ( 'NONE',  ( -13.91746824999999532, 79.27500000273117564, -4.522059556121115875 ) ) ;
#30368=CARTESIAN_POINT ( 'NONE',  ( -9.270509831248421762, 76.55000000546237970, 12.75976212528060039 ) ) ;
#30380=CARTESIAN_POINT ( 'NONE',  ( -4.300734207923759378, 80.97500000273122112, -13.23629886949340495 ) ) ;
#30384=CARTESIAN_POINT ( 'NONE',  ( 15.00000000000000355, 78.90000000000000568, 4.873795443493592394 ) ) ;
#30434=ORIENTED_EDGE ( 'NONE', *, *, #19726, .T. ) ;
#30440=VECTOR ( 'NONE', #31100, 1000.000000000000000 ) ;
#30441=CARTESIAN_POINT ( 'NONE',  ( -12.13525491562421088, 75.80000000000003979, -8.816778784387096835 ) ) ;
#30457=CARTESIAN_POINT ( 'NONE',  ( 4.300734207923761154, 71.47500000273116427, 13.23629886949340495 ) ) ;
#30475=ORIENTED_EDGE ( 'NONE', *, *, #6564, .T. ) ;
#30485=CARTESIAN_POINT ( 'NONE',  ( -13.62972974288548933, 74.00000000000002842, 5.724431369363315092 ) ) ;
#30490=AXIS2_PLACEMENT_3D ( 'NONE', #8686, #19170, #1973 ) ;
#30523=AXIS2_PLACEMENT_3D ( 'NONE', #17538, #4657, #9808 ) ;
#30525=CARTESIAN_POINT ( 'NONE',  ( 9.270509831248421762, 79.55000000546240813, -12.75976212528059861 ) ) ;
#30529=CARTESIAN_POINT ( 'NONE',  ( 4.635254915624209993, 81.39999999999997726, -14.26584774442730463 ) ) ;
#30541=CARTESIAN_POINT ( 'NONE',  ( 9.270509831248423538, 77.55000000546233707, -12.75976212528059861 ) ) ;
#30552=CARTESIAN_POINT ( 'NONE',  ( -8.601468415847518756, 80.57500000273120122, -11.83890561707634603 ) ) ;
#30555=CARTESIAN_POINT ( 'NONE',  ( 4.300734207923757602, 74.27500000273118985, -13.23629886949340673 ) ) ;
#30611=DIRECTION ( 'NONE',  ( 0.000000000000000000, -0.000000000000000000, 1.000000000000000000 ) ) ;
#30627=CARTESIAN_POINT ( 'NONE',  ( 15.00000000000000355, 74.90000000000001990, 4.873795443493592394 ) ) ;
#30657=CARTESIAN_POINT ( 'NONE',  ( -13.75194420523858341, 74.00000000000004263, 5.454580986648785768 ) ) ;
#30701=CARTESIAN_POINT ( 'NONE',  ( -15.00000000000000000, 79.89999999999997726, -4.873795443493594171 ) ) ;
#30714=CARTESIAN_POINT ( 'NONE',  ( -9.657523855033125146E-16, 77.75000000546233991, -15.77193336357400710 ) ) ;
#30727=CARTESIAN_POINT ( 'NONE',  ( -13.91746824999999887, 74.87500000273116996, 0.000000000000000000 ) ) ;
#30738=EDGE_CURVE ( 'NONE', #30951, #13542, #26773, .T. ) ;
#30831=EDGE_CURVE ( 'NONE', #8605, #21926, #23218, .T. ) ;
#30835=CARTESIAN_POINT ( 'NONE',  ( -13.22843218963023837, 74.00000000000005684, 6.523198192541685536 ) ) ;
#30875=CARTESIAN_POINT ( 'NONE',  ( -9.270509831248425314, 75.69999999999998863, -12.75976212528059861 ) ) ;
#30888=CARTESIAN_POINT ( 'NONE',  ( 12.13525491562420910, 79.45000000546237118, -8.816778784387098611 ) ) ;
#30903=CARTESIAN_POINT ( 'NONE',  ( -8.601468415847515203, 75.17500000273118133, 11.83890561707634959 ) ) ;
#30908=CARTESIAN_POINT ( 'NONE',  ( 15.00000000000000000, 79.10000000000000853, -4.873795443493596835 ) ) ;
#30951=VERTEX_POINT ( 'NONE', #9584 ) ;
#30953=CARTESIAN_POINT ( 'NONE',  ( 0.000000000000000000, 74.00000000000001421, 0.000000000000000000 ) ) ;
#30956=ORIENTED_EDGE ( 'NONE', *, *, #28553, .F. ) ;
#31025=( BOUNDED_SURFACE ( )  B_SPLINE_SURFACE ( 1, 2, ( 
 ( #32772, #7037, #9266, #3959, #22486, #14433, #9614, #12188, #30888, #14942, #7209, #33112, #14603, #27981, #25060, #24888, #22831, #9435, #9789, #19920, #12363, #17348, #20096, #33291, #1372, #30714, #1541, #30541, #22327, #12017, #17520, #7384, #1710, #32937, #27811, #11848, #17868, #30368, #17692, #4468, #28152, #19750, #20267, #4295, #30198, #25407, #17182, #22658, #4638, #1885, #14770, #25235, #6699, #15117, #25581, #2061, #12537, #23006, #27640, #33463, #4128, #9963, #20438, #5787, #21082, #18679, #32027, #8690, #8189, #24319, #10775, #13524, #33639, #13853, #5622, #29119, #23987, #3220, #25747, #21581, #26389, #21416, #12706, #2882, #10941, #21751, #26557, #13348, #31696, #4808, #32196, #287, #8524, #31859, #19008, #10604, #24152, #5452, #28320, #29287, #8024 ),
 ( #23821, #18510, #18841, #11112, #21252, #15287, #2229, #792, #16268, #8352, #11275, #29452, #5954, #31531, #16434, #459, #16106, #3053, #23177, #26725, #15933, #13688, #26886, #623, #3383, #28956, #4043, #16596, #22406, #6113, #19505, #29780, #32854, #24639, #24479, #6456, #30285, #16930, #27051, #1113, #9349, #3877, #17097, #9023, #3544, #3713, #14016, #1624, #25148, #6786, #11433, #27555, #953, #12102, #14517, #14183, #21910, #14350, #17264, #22246, #6285, #6618, #24976, #1285, #11598, #29952, #22079, #24807, #32523, #1459, #27388, #11764, #32360, #11937, #8854, #19336, #32690, #19174, #16761, #19832, #27727, #27220, #4215, #22573, #9185, #19669, #14689, #30114, #33024, #29611, #33733, #12967, #15033, #25323, #30457, #9875, #20710, #1798, #20183, #12797, #6954 ) ),
 .UNSPECIFIED., .F., .F., .T. ) 
 B_SPLINE_SURFACE_WITH_KNOTS ( ( 2, 2 ),
 ( 3, 2, 2, 2, 2, 2, 2, 2, 2, 2, 2, 2, 2, 2, 2, 2, 2, 2, 2, 2, 2, 2, 2, 2, 2, 2, 2, 2, 2, 2, 2, 2, 2, 2, 2, 2, 2, 2, 2, 2, 2, 2, 2, 2, 2, 2, 2, 2, 2, 2, 3 ),
 ( 0.000000000000000000, 1.000000000000000000 ),
 ( 0.000000000000000000, 0.02000000000000000042, 0.04000000000000000083, 0.05999999999999999778, 0.08000000000000000167, 0.1000000000000000056, 0.1199999999999999956, 0.1400000000000000133, 0.1600000000000000033, 0.1799999999999999933, 0.2000000000000000111, 0.2200000000000000011, 0.2399999999999999911, 0.2600000000000000089, 0.2800000000000000266, 0.2999999999999999889, 0.3200000000000000067, 0.3400000000000000244, 0.3599999999999999867, 0.3800000000000000044, 0.4000000000000000222, 0.4199999999999999845, 0.4400000000000000022, 0.4600000000000000200, 0.4799999999999999822, 0.5000000000000000000, 0.5200000000000000178, 0.5400000000000000355, 0.5600000000000000533, 0.5799999999999999600, 0.5999999999999999778, 0.6199999999999999956, 0.6400000000000000133, 0.6600000000000000311, 0.6800000000000000488, 0.6999999999999999556, 0.7199999999999999734, 0.7399999999999999911, 0.7600000000000000089, 0.7800000000000000266, 0.8000000000000000444, 0.8199999999999999512, 0.8399999999999999689, 0.8599999999999999867, 0.8800000000000000044, 0.9000000000000000222, 0.9200000000000000400, 0.9399999999999999467, 0.9599999999999999645, 0.9799999999999999822, 1.000000000000000000 ),
 .UNSPECIFIED. ) 
 GEOMETRIC_REPRESENTATION_ITEM ( )  RATIONAL_B_SPLINE_SURFACE ( (
 ( 1.000000000000000000, 0.9510565162951535312, 1.000000000000000000, 0.9510565162951535312, 1.000000000000000000, 0.9510565162951535312, 1.000000000000000000, 0.9510565162951535312, 1.000000000000000000, 0.9510565162951535312, 1.000000000000000000, 0.9510565162951535312, 1.000000000000000000, 0.9510565162951535312, 1.000000000000000000, 0.9510565162951535312, 1.000000000000000000, 0.9510565162951535312, 1.000000000000000000, 0.9510565162951535312, 1.000000000000000000, 0.9510565162951535312, 1.000000000000000000, 0.9510565162951535312, 1.000000000000000000, 0.9510565162951535312, 1.000000000000000000, 0.9510565162951535312, 1.000000000000000000, 0.9510565162951535312, 1.000000000000000000, 0.9510565162951535312, 1.000000000000000000, 0.9510565162951535312, 1.000000000000000000, 0.9510565162951535312, 1.000000000000000000, 0.9510565162951535312, 1.000000000000000000, 0.9510565162951535312, 1.000000000000000000, 0.9510565162951535312, 1.000000000000000000, 0.9510565162951535312, 1.000000000000000000, 0.9510565162951535312, 1.000000000000000000, 0.9510565162951535312, 1.000000000000000000, 0.9510565162951535312, 1.000000000000000000, 0.9510565162951535312, 1.000000000000000000, 0.9510565162951535312, 1.000000000000000000, 0.9510565162951535312, 1.000000000000000000, 0.9510565162951535312, 1.000000000000000000, 0.9510565162951535312, 1.000000000000000000, 0.9510565162951535312, 1.000000000000000000, 0.9510565162951535312, 1.000000000000000000, 0.9510565162951535312, 1.000000000000000000, 0.9510565162951535312, 1.000000000000000000, 0.9510565162951535312, 1.000000000000000000, 0.9510565162951535312, 1.000000000000000000, 0.9510565162951535312, 1.000000000000000000, 0.9510565162951535312, 1.000000000000000000, 0.9510565162951535312, 1.000000000000000000, 0.9510565162951535312, 1.000000000000000000, 0.9510565162951535312, 1.000000000000000000, 0.9510565162951535312, 1.000000000000000000, 0.9510565162951535312, 1.000000000000000000, 0.9510565162951535312, 1.000000000000000000, 0.9510565162951535312, 1.000000000000000000, 0.9510565162951535312, 1.000000000000000000, 0.9510565162951535312, 1.000000000000000000, 0.9510565162951535312, 1.000000000000000000, 0.9510565162951535312, 1.000000000000000000, 0.9510565162951535312, 1.000000000000000000),
 ( 1.000000000000000000, 0.9510565162951535312, 1.000000000000000000, 0.9510565162951535312, 1.000000000000000000, 0.9510565162951535312, 1.000000000000000000, 0.9510565162951535312, 1.000000000000000000, 0.9510565162951535312, 1.000000000000000000, 0.9510565162951535312, 1.000000000000000000, 0.9510565162951535312, 1.000000000000000000, 0.9510565162951535312, 1.000000000000000000, 0.9510565162951535312, 1.000000000000000000, 0.9510565162951535312, 1.000000000000000000, 0.9510565162951535312, 1.000000000000000000, 0.9510565162951535312, 1.000000000000000000, 0.9510565162951535312, 1.000000000000000000, 0.9510565162951535312, 1.000000000000000000, 0.9510565162951535312, 1.000000000000000000, 0.9510565162951535312, 1.000000000000000000, 0.9510565162951535312, 1.000000000000000000, 0.9510565162951535312, 1.000000000000000000, 0.9510565162951535312, 1.000000000000000000, 0.9510565162951535312, 1.000000000000000000, 0.9510565162951535312, 1.000000000000000000, 0.9510565162951535312, 1.000000000000000000, 0.9510565162951535312, 1.000000000000000000, 0.9510565162951535312, 1.000000000000000000, 0.9510565162951535312, 1.000000000000000000, 0.9510565162951535312, 1.000000000000000000, 0.9510565162951535312, 1.000000000000000000, 0.9510565162951535312, 1.000000000000000000, 0.9510565162951535312, 1.000000000000000000, 0.9510565162951535312, 1.000000000000000000, 0.9510565162951535312, 1.000000000000000000, 0.9510565162951535312, 1.000000000000000000, 0.9510565162951535312, 1.000000000000000000, 0.9510565162951535312, 1.000000000000000000, 0.9510565162951535312, 1.000000000000000000, 0.9510565162951535312, 1.000000000000000000, 0.9510565162951535312, 1.000000000000000000, 0.9510565162951535312, 1.000000000000000000, 0.9510565162951535312, 1.000000000000000000, 0.9510565162951535312, 1.000000000000000000, 0.9510565162951535312, 1.000000000000000000, 0.9510565162951535312, 1.000000000000000000, 0.9510565162951535312, 1.000000000000000000, 0.9510565162951535312, 1.000000000000000000, 0.9510565162951535312, 1.000000000000000000, 0.9510565162951535312, 1.000000000000000000, 0.9510565162951535312, 1.000000000000000000, 0.9510565162951535312, 1.000000000000000000, 0.9510565162951535312, 1.000000000000000000, 0.9510565162951535312, 1.000000000000000000) ) ) 
 REPRESENTATION_ITEM ( '' )  SURFACE ( )  );
#31041=DIRECTION ( 'NONE',  ( 0.000000000000000000, 1.000000000000000000, 0.000000000000000000 ) ) ;
#31049=AXIS2_PLACEMENT_3D ( 'NONE', #12270, #22744, #33547 ) ;
#31052=CARTESIAN_POINT ( 'NONE',  ( -9.270509831248421762, 78.29999999999995453, 12.75976212528060039 ) ) ;
#31071=VECTOR ( 'NONE', #12458, 1000.000000000000000 ) ;
#31075=CARTESIAN_POINT ( 'NONE',  ( -11.25946833292375793, 79.17500000273119554, -8.180482586598733619 ) ) ;
#31100=DIRECTION ( 'NONE',  ( -3.169619151431772337E-17, -0.9659258262890680902, -0.2588190451025213501 ) ) ;
#31104=DIRECTION ( 'NONE',  ( 0.4999999999999996114, 0.000000000000000000, -0.8660254037844388186 ) ) ;
#31152=CARTESIAN_POINT ( 'NONE',  ( 2.375766604868043252, 75.44874571845315359, -14.99999999999999822 ) ) ;
#31175=EDGE_CURVE ( 'NONE', #9461, #29890, #11700, .T. ) ;
#31180=CARTESIAN_POINT ( 'NONE',  ( 0.000000000000000000, 102.0000000000000284, 0.000000000000000000 ) ) ;
#31183=CARTESIAN_POINT ( 'NONE',  ( 1.102182119232617911E-15, 122.0000000000000000, 9.000000000000001776 ) ) ;
#31209=ORIENTED_EDGE ( 'NONE', *, *, #9244, .F. ) ;
#31216=CARTESIAN_POINT ( 'NONE',  ( 2.375766604868044141, 79.69874572391552192, -14.99999999999999822 ) ) ;
#31219=CARTESIAN_POINT ( 'NONE',  ( -15.00000000000000000, 78.09999999999999432, 4.873795443493597723 ) ) ;
#31240=CARTESIAN_POINT ( 'NONE',  ( 8.601468415847516980, 74.17500000273122396, -11.83890561707634603 ) ) ;
#31243=CARTESIAN_POINT ( 'NONE',  ( 8.601468415847520532, 76.07500000273115859, 11.83890561707634781 ) ) ;
#31260=CARTESIAN_POINT ( 'NONE',  ( -12.13525491562421088, 76.05000000546240813, -8.816778784387096835 ) ) ;
#31293=CIRCLE ( 'NONE', #15978, 9.000000000000001776 ) ;
#31309=CARTESIAN_POINT ( 'NONE',  ( 15.00000000000000000, 81.09999999999999432, -4.873795443493596835 ) ) ;
#31389=CARTESIAN_POINT ( 'NONE',  ( -15.00000000000000000, 74.00000000000001421, 0.000000000000000000 ) ) ;
#31392=CARTESIAN_POINT ( 'NONE',  ( 11.54700538379251817, 96.00000000000002842, 19.99999999999999645 ) ) ;
#31411=CARTESIAN_POINT ( 'NONE',  ( -8.960552108402744065E-16, 76.37500000273114154, -14.63369212191046209 ) ) ;
#31414=CARTESIAN_POINT ( 'NONE',  ( 4.300734207923761154, 73.97500000273122112, 13.23629886949340495 ) ) ;
#31433=DIRECTION ( 'NONE',  ( -0.000000000000000000, -1.000000000000000000, -0.000000000000000000 ) ) ;
#31465=CARTESIAN_POINT ( 'NONE',  ( -8.891200544363830713E-16, 77.49999999999998579, -15.00000000000000000 ) ) ;
#31476=CARTESIAN_POINT ( 'NONE',  ( 0.000000000000000000, 74.00000000000001421, 0.000000000000000000 ) ) ;
#31478=STYLED_ITEM ( 'NONE', ( #11632 ), #29162 ) ;
#31508=ORIENTED_EDGE ( 'NONE', *, *, #3277, .F. ) ;
#31531=CARTESIAN_POINT ( 'NONE',  ( 8.601468415847520532, 79.57500000273117280, 11.83890561707634781 ) ) ;
#31563=CARTESIAN_POINT ( 'NONE',  ( -10.14794146028621924, 74.00000000000002842, -11.03244795973553849 ) ) ;
#31573=CARTESIAN_POINT ( 'NONE',  ( -13.91746824999999887, 76.87500000273116996, 0.000000000000000000 ) ) ;
#31576=CARTESIAN_POINT ( 'NONE',  ( 4.300734207923757602, 78.77500000273118985, -13.23629886949340673 ) ) ;
#31596=EDGE_CURVE ( 'NONE', #871, #30951, #24123, .T. ) ;
#31665=VECTOR ( 'NONE', #26054, 1000.000000000000000 ) ;
#31696=CARTESIAN_POINT ( 'NONE',  ( 12.13525491562420910, 71.45000000546237118, -8.816778784387098611 ) ) ;
#31725=CARTESIAN_POINT ( 'NONE',  ( -4.223320258572821363E-15, 78.75000000546236834, 15.00000000000000355 ) ) ;
#31732=CARTESIAN_POINT ( 'NONE',  ( 9.930763101775172075, 74.00000000000000000, -10.06536667093442006 ) ) ;
#31742=DIRECTION ( 'NONE',  ( 0.000000000000000000, 0.000000000000000000, 1.000000000000000000 ) ) ;
#31743=CARTESIAN_POINT ( 'NONE',  ( 13.91746824999999887, 75.87500000273116996, -1.704398294459741270E-15 ) ) ;
#31746=CARTESIAN_POINT ( 'NONE',  ( 2.688165632520823219E-15, 73.87500000273116996, 14.63369212191046387 ) ) ;
#31760=CARTESIAN_POINT ( 'NONE',  ( 11.25946833292375793, 76.17500000273119554, 8.180482586598731842 ) ) ;
#31797=ORIENTED_EDGE ( 'NONE', *, *, #17545, .T. ) ;
#31836=ORIENTED_EDGE ( 'NONE', *, *, #21746, .T. ) ;
#31859=CARTESIAN_POINT ( 'NONE',  ( 9.270509831248425314, 70.95000000546237118, 12.75976212528059683 ) ) ;
#31864=CARTESIAN_POINT ( 'NONE',  ( -12.13525491562421088, 80.05000000546236549, -8.816778784387096835 ) ) ;
#31865=CARTESIAN_POINT ( 'NONE',  ( -2.375766604868044585, 80.44874571845313938, 14.99999999999999822 ) ) ;
#31895=CARTESIAN_POINT ( 'NONE',  ( -8.219587594935800823, 74.00000000000002842, -12.42830407035704177 ) ) ;
#31903=PRODUCT_DEFINITION_CONTEXT ( 'detailed design', #14461, 'design' ) ;
#31907=CARTESIAN_POINT ( 'NONE',  ( -8.960552108402744065E-16, 78.37500000273119838, -14.63369212191046209 ) ) ;
#31910=CARTESIAN_POINT ( 'NONE',  ( 2.688165632520823219E-15, 71.87500000273116996, 14.63369212191046387 ) ) ;
#31918=( BOUNDED_SURFACE ( )  B_SPLINE_SURFACE ( 1, 2, ( 
 ( #18909, #16334, #11010, #858, #29355, #11177, #5691, #16664, #8755, #5856, #26790, #11338, #13591, #3282, #16494, #13750, #5521, #24220, #691, #32095, #24055, #26948, #8590, #18578, #21814, #13918, #32263, #19239, #18744, #19075, #6182, #21480, #523, #29514, #26625, #24385, #8091, #29677, #29186, #2777, #29019, #2947, #357, #13241, #23716, #10671, #21150, #16000, #26456, #23886, #10841, #21319, #31760, #8251, #16169, #3120, #31927, #6858, #17337, #32427, #14758, #19739, #6526, #22475, #22315, #1358, #3781, #12004, #30356, #32923, #16999, #27800, #9422, #24545, #4284, #14088, #27456, #14252, #25221, #32593, #8923, #19406, #22149, #6355, #30184, #6687, #1699, #12176, #16834, #1530, #9092, #1186, #33100, #17171, #19907, #27628, #24876, #11837, #19574, #22647, #11499 ),
 ( #27289, #9603, #1016, #32760, #20085, #29854, #30529, #7026, #21978, #27121, #3614, #24709, #4116, #3947, #14590, #11668, #25049, #30022, #14422, #9254, #10125, #30701, #7372, #4971, #20257, #12694, #13039, #7197, #26077, #25396, #23164, #23343, #33279, #15626, #33805, #9775, #12865, #31052, #2215, #31219, #28140, #20607, #20426, #10462, #12351, #20940, #17678, #9951, #4626, #15105, #28475, #18029, #7544, #2397, #15448, #33626, #25570, #33452, #4453, #2050, #4796, #25903, #12525, #30875, #22993, #10298, #17856, #25736, #18199, #20775, #28308, #2573, #7712, #28642, #15275, #1873, #22820, #5138, #23510, #33968, #31389, #17509, #27970, #14930, #18537, #26752, #15793, #15960, #24014, #11140, #8382, #8051, #10802, #28814, #13551, #28983, #23850, #3245, #651, #142, #486 ) ),
 .UNSPECIFIED., .F., .F., .T. ) 
 B_SPLINE_SURFACE_WITH_KNOTS ( ( 2, 2 ),
 ( 3, 2, 2, 2, 2, 2, 2, 2, 2, 2, 2, 2, 2, 2, 2, 2, 2, 2, 2, 2, 2, 2, 2, 2, 2, 2, 2, 2, 2, 2, 2, 2, 2, 2, 2, 2, 2, 2, 2, 2, 2, 2, 2, 2, 2, 2, 2, 2, 2, 2, 3 ),
 ( 0.000000000000000000, 1.000000000000000000 ),
 ( 0.000000000000000000, 0.02000000000000000042, 0.04000000000000000083, 0.05999999999999999778, 0.08000000000000000167, 0.1000000000000000056, 0.1199999999999999956, 0.1400000000000000133, 0.1600000000000000033, 0.1799999999999999933, 0.2000000000000000111, 0.2200000000000000011, 0.2399999999999999911, 0.2600000000000000089, 0.2800000000000000266, 0.2999999999999999889, 0.3200000000000000067, 0.3400000000000000244, 0.3599999999999999867, 0.3800000000000000044, 0.4000000000000000222, 0.4199999999999999845, 0.4400000000000000022, 0.4600000000000000200, 0.4799999999999999822, 0.5000000000000000000, 0.5200000000000000178, 0.5400000000000000355, 0.5600000000000000533, 0.5799999999999999600, 0.5999999999999999778, 0.6199999999999999956, 0.6400000000000000133, 0.6600000000000000311, 0.6800000000000000488, 0.6999999999999999556, 0.7199999999999999734, 0.7399999999999999911, 0.7600000000000000089, 0.7800000000000000266, 0.8000000000000000444, 0.8199999999999999512, 0.8399999999999999689, 0.8599999999999999867, 0.8800000000000000044, 0.9000000000000000222, 0.9200000000000000400, 0.9399999999999999467, 0.9599999999999999645, 0.9799999999999999822, 1.000000000000000000 ),
 .UNSPECIFIED. ) 
 GEOMETRIC_REPRESENTATION_ITEM ( )  RATIONAL_B_SPLINE_SURFACE ( (
 ( 1.000000000000000000, 0.9510565162951535312, 1.000000000000000000, 0.9510565162951535312, 1.000000000000000000, 0.9510565162951535312, 1.000000000000000000, 0.9510565162951535312, 1.000000000000000000, 0.9510565162951535312, 1.000000000000000000, 0.9510565162951535312, 1.000000000000000000, 0.9510565162951535312, 1.000000000000000000, 0.9510565162951535312, 1.000000000000000000, 0.9510565162951535312, 1.000000000000000000, 0.9510565162951535312, 1.000000000000000000, 0.9510565162951535312, 1.000000000000000000, 0.9510565162951535312, 1.000000000000000000, 0.9510565162951535312, 1.000000000000000000, 0.9510565162951535312, 1.000000000000000000, 0.9510565162951535312, 1.000000000000000000, 0.9510565162951535312, 1.000000000000000000, 0.9510565162951535312, 1.000000000000000000, 0.9510565162951535312, 1.000000000000000000, 0.9510565162951535312, 1.000000000000000000, 0.9510565162951535312, 1.000000000000000000, 0.9510565162951535312, 1.000000000000000000, 0.9510565162951535312, 1.000000000000000000, 0.9510565162951535312, 1.000000000000000000, 0.9510565162951535312, 1.000000000000000000, 0.9510565162951535312, 1.000000000000000000, 0.9510565162951535312, 1.000000000000000000, 0.9510565162951535312, 1.000000000000000000, 0.9510565162951535312, 1.000000000000000000, 0.9510565162951535312, 1.000000000000000000, 0.9510565162951535312, 1.000000000000000000, 0.9510565162951535312, 1.000000000000000000, 0.9510565162951535312, 1.000000000000000000, 0.9510565162951535312, 1.000000000000000000, 0.9510565162951535312, 1.000000000000000000, 0.9510565162951535312, 1.000000000000000000, 0.9510565162951535312, 1.000000000000000000, 0.9510565162951535312, 1.000000000000000000, 0.9510565162951535312, 1.000000000000000000, 0.9510565162951535312, 1.000000000000000000, 0.9510565162951535312, 1.000000000000000000, 0.9510565162951535312, 1.000000000000000000, 0.9510565162951535312, 1.000000000000000000, 0.9510565162951535312, 1.000000000000000000, 0.9510565162951535312, 1.000000000000000000, 0.9510565162951535312, 1.000000000000000000, 0.9510565162951535312, 1.000000000000000000, 0.9510565162951535312, 1.000000000000000000, 0.9510565162951535312, 1.000000000000000000, 0.9510565162951535312, 1.000000000000000000, 0.9510565162951535312, 1.000000000000000000),
 ( 1.000000000000000000, 0.9510565162951535312, 1.000000000000000000, 0.9510565162951535312, 1.000000000000000000, 0.9510565162951535312, 1.000000000000000000, 0.9510565162951535312, 1.000000000000000000, 0.9510565162951535312, 1.000000000000000000, 0.9510565162951535312, 1.000000000000000000, 0.9510565162951535312, 1.000000000000000000, 0.9510565162951535312, 1.000000000000000000, 0.9510565162951535312, 1.000000000000000000, 0.9510565162951535312, 1.000000000000000000, 0.9510565162951535312, 1.000000000000000000, 0.9510565162951535312, 1.000000000000000000, 0.9510565162951535312, 1.000000000000000000, 0.9510565162951535312, 1.000000000000000000, 0.9510565162951535312, 1.000000000000000000, 0.9510565162951535312, 1.000000000000000000, 0.9510565162951535312, 1.000000000000000000, 0.9510565162951535312, 1.000000000000000000, 0.9510565162951535312, 1.000000000000000000, 0.9510565162951535312, 1.000000000000000000, 0.9510565162951535312, 1.000000000000000000, 0.9510565162951535312, 1.000000000000000000, 0.9510565162951535312, 1.000000000000000000, 0.9510565162951535312, 1.000000000000000000, 0.9510565162951535312, 1.000000000000000000, 0.9510565162951535312, 1.000000000000000000, 0.9510565162951535312, 1.000000000000000000, 0.9510565162951535312, 1.000000000000000000, 0.9510565162951535312, 1.000000000000000000, 0.9510565162951535312, 1.000000000000000000, 0.9510565162951535312, 1.000000000000000000, 0.9510565162951535312, 1.000000000000000000, 0.9510565162951535312, 1.000000000000000000, 0.9510565162951535312, 1.000000000000000000, 0.9510565162951535312, 1.000000000000000000, 0.9510565162951535312, 1.000000000000000000, 0.9510565162951535312, 1.000000000000000000, 0.9510565162951535312, 1.000000000000000000, 0.9510565162951535312, 1.000000000000000000, 0.9510565162951535312, 1.000000000000000000, 0.9510565162951535312, 1.000000000000000000, 0.9510565162951535312, 1.000000000000000000, 0.9510565162951535312, 1.000000000000000000, 0.9510565162951535312, 1.000000000000000000, 0.9510565162951535312, 1.000000000000000000, 0.9510565162951535312, 1.000000000000000000, 0.9510565162951535312, 1.000000000000000000, 0.9510565162951535312, 1.000000000000000000, 0.9510565162951535312, 1.000000000000000000, 0.9510565162951535312, 1.000000000000000000) ) ) 
 REPRESENTATION_ITEM ( '' )  SURFACE ( )  );
#31924=DIRECTION ( 'NONE',  ( -0.4999999999999997224, 0.000000000000000000, 0.8660254037844388186 ) ) ;
#31927=CARTESIAN_POINT ( 'NONE',  ( -4.300734207923755825, 75.77500000273118985, 13.23629886949340673 ) ) ;
#31929=CARTESIAN_POINT ( 'NONE',  ( -8.891200544363830713E-16, 75.50000000000000000, -15.00000000000000000 ) ) ;
#31931=DIRECTION ( 'NONE',  ( 0.000000000000000000, 0.000000000000000000, 1.000000000000000000 ) ) ;
#31941=CONICAL_SURFACE ( 'NONE', #7845, 13.32050807568876927, 0.2617993877991500740 ) ;
#31954=CARTESIAN_POINT ( 'NONE',  ( 8.601468415847516980, 76.17500000273115290, -11.83890561707634781 ) ) ;
#32027=CARTESIAN_POINT ( 'NONE',  ( 4.635254915624209993, 73.65000000546240244, -14.26584774442730463 ) ) ;
#32033=CARTESIAN_POINT ( 'NONE',  ( -4.635254915624211769, 79.60000000000000853, -14.26584774442730286 ) ) ;
#32042=ORIENTED_EDGE ( 'NONE', *, *, #18121, .F. ) ;
#32070=MANIFOLD_SOLID_BREP ( 'Cavity1', #1300 ) ;
#32079=AXIS2_PLACEMENT_3D ( 'NONE', #16005, #23554, #11014 ) ;
#32080=DIRECTION ( 'NONE',  ( -0.000000000000000000, 1.000000000000000000, -0.000000000000000000 ) ) ;
#32095=CARTESIAN_POINT ( 'NONE',  ( -13.91746824999999532, 79.47500000273115006, 4.522059556121122093 ) ) ;
#32121=CARTESIAN_POINT ( 'NONE',  ( 13.91746824999999887, 79.87500000273118417, -1.704398294459741270E-15 ) ) ;
#32162=DIRECTION ( 'NONE',  ( 0.000000000000000000, 0.000000000000000000, 1.000000000000000000 ) ) ;
#32196=CARTESIAN_POINT ( 'NONE',  ( 15.00000000000000000, 71.25000000546238255, -1.836970198721029589E-15 ) ) ;
#32216=EDGE_CURVE ( 'NONE', #9461, #23625, #6168, .T. ) ;
#32263=CARTESIAN_POINT ( 'NONE',  ( 4.300734207923757602, 78.77500000273118985, -13.23629886949340673 ) ) ;
#32271=CARTESIAN_POINT ( 'NONE',  ( 13.91746824999999532, 78.47500000273120691, -4.522059556121118540 ) ) ;
#32275=ORIENTED_EDGE ( 'NONE', *, *, #15946, .F. ) ;
#32278=DIRECTION ( 'NONE',  ( 0.000000000000000000, 1.000000000000000000, 0.000000000000000000 ) ) ;
#32286=CARTESIAN_POINT ( 'NONE',  ( 8.601468415847516980, 78.17500000273120975, -11.83890561707634781 ) ) ;
#32290=ORIENTED_EDGE ( 'NONE', *, *, #7128, .F. ) ;
#32299=ORIENTED_EDGE ( 'NONE', *, *, #9790, .F. ) ;
#32316=ORIENTED_EDGE ( 'NONE', *, *, #4738, .T. ) ;
#32344=CARTESIAN_POINT ( 'NONE',  ( -8.891200544363830713E-16, 75.75000000546238255, -15.00000000000000000 ) ) ;
#32360=CARTESIAN_POINT ( 'NONE',  ( 11.25946833292375793, 73.67500000273119554, 8.180482586598731842 ) ) ;
#32365=CARTESIAN_POINT ( 'NONE',  ( -15.00000000000000000, 80.25000000546239676, 0.000000000000000000 ) ) ;
#32395=VECTOR ( 'NONE', #12893, 1000.000000000000000 ) ;
#32427=CARTESIAN_POINT ( 'NONE',  ( -13.91746824999999532, 75.47500000273116427, 4.522059556121122093 ) ) ;
#32436=CARTESIAN_POINT ( 'NONE',  ( -11.25946833292375793, 79.57500000273121543, 8.180482586598737171 ) ) ;
#32440=ORIENTED_EDGE ( 'NONE', *, *, #21679, .T. ) ;
#32451=CARTESIAN_POINT ( 'NONE',  ( -13.91746824999999532, 80.77500000273118985, -4.522059556121115875 ) ) ;
#32462=EDGE_LOOP ( 'NONE', ( #9164, #18426, #33443, #12513 ) ) ;
#32475=CARTESIAN_POINT ( 'NONE',  ( 0.000000000000000000, 122.0000000000000000, 0.000000000000000000 ) ) ;
#32523=CARTESIAN_POINT ( 'NONE',  ( 11.25946833292375793, 74.07500000273120122, -8.180482586598735395 ) ) ;
#32593=CARTESIAN_POINT ( 'NONE',  ( -13.91746824999999532, 73.47500000273117848, 4.522059556121122093 ) ) ;
#32603=CARTESIAN_POINT ( 'NONE',  ( 13.91746824999999532, 76.47500000273120691, -4.522059556121118540 ) ) ;
#32650=PLANE ( 'NONE',  #1368 ) ;
#32674=CARTESIAN_POINT ( 'NONE',  ( -9.270509831248423538, 75.69999999999998863, -12.75976212528059861 ) ) ;
#32690=CARTESIAN_POINT ( 'NONE',  ( -4.300734207923755825, 73.27500000273118985, 13.23629886949340673 ) ) ;
#32700=CARTESIAN_POINT ( 'NONE',  ( -9.270509831248423538, 77.69999999999998863, -12.75976212528059861 ) ) ;
#32719=CARTESIAN_POINT ( 'NONE',  ( 4.805950183054497948, 74.00000000000001421, 13.09988514501729284 ) ) ;
#32724=( NAMED_UNIT ( * ) SI_UNIT ( $, .STERADIAN. ) SOLID_ANGLE_UNIT ( ) );
#32741=CARTESIAN_POINT ( 'NONE',  ( -2.375766604868045029, 77.80125428700921475, -14.99999999999999822 ) ) ;
#32760=CARTESIAN_POINT ( 'NONE',  ( -9.270509831248425314, 81.69999999999998863, -12.75976212528059861 ) ) ;
#32769=CARTESIAN_POINT ( 'NONE',  ( 23.09401076758502569, 86.00000000000001421, -6.857326241137392698E-15 ) ) ;
#32770=CARTESIAN_POINT ( 'NONE',  ( 13.91746824999999887, 78.37500000273116996, -1.704398294459741270E-15 ) ) ;
#32772=CARTESIAN_POINT ( 'NONE',  ( -15.00000000000000000, 80.25000000546239676, 0.000000000000000000 ) ) ;
#32776=CARTESIAN_POINT ( 'NONE',  ( -4.635254915624208216, 74.65000000546240244, 14.26584774442730463 ) ) ;
#32785=CARTESIAN_POINT ( 'NONE',  ( 4.300734207923761154, 73.47500000273116427, 13.23629886949340495 ) ) ;
#32834=ORIENTED_EDGE ( 'NONE', *, *, #10703, .F. ) ;
#32836=CARTESIAN_POINT ( 'NONE',  ( -15.00000000000010125, 74.09999999999999432, 4.873795443493460944 ) ) ;
#32840=CARTESIAN_POINT ( 'NONE',  ( -2.375766604868045029, 75.55125428154684641, -14.99999999999999822 ) ) ;
#32854=CARTESIAN_POINT ( 'NONE',  ( 11.25946833292375793, 77.67500000273119554, 8.180482586598731842 ) ) ;
#32882=CARTESIAN_POINT ( 'NONE',  ( -14.97879338252777259, 74.00000000000004263, 0.5967302757886839837 ) ) ;
#32923=CARTESIAN_POINT ( 'NONE',  ( 13.91746824999999532, 74.47500000273120691, -4.522059556121118540 ) ) ;
#32935=CARTESIAN_POINT ( 'NONE',  ( -8.601468415847518756, 79.07500000273118701, -11.83890561707634603 ) ) ;
#32937=CARTESIAN_POINT ( 'NONE',  ( 9.270509831248425314, 76.95000000546237118, 12.75976212528059683 ) ) ;
#32948=CARTESIAN_POINT ( 'NONE',  ( -11.25946833292375793, 73.07500000273120122, 8.180482586598737171 ) ) ;
#32981=CARTESIAN_POINT ( 'NONE',  ( 23.09401076758502569, 96.00000000000002842, -6.857326241137392698E-15 ) ) ;
#32992=DIRECTION ( 'NONE',  ( 0.000000000000000000, -0.000000000000000000, 1.000000000000000000 ) ) ;
#32996=VECTOR ( 'NONE', #6668, 1000.000000000000000 ) ;
#33004=( BOUNDED_CURVE ( )  B_SPLINE_CURVE ( 2, ( #24554, #16843, #3624, #14098, #1370, #24886, #3957, #19748, #14431, #30031, #21988, #6365, #11347, #8935, #11677, #11846, #19415, #3791, #32436, #9102, #1027, #30366, #27299, #32935, #11508, #27638, #22325, #6192, #9433, #32271, #32770, #14262, #29864, #6536, #19583, #19247, #30196, #19918, #24720, #17009, #29686, #6697, #1196, #14601, #17180, #8764, #25058, #16673, #22160, #32603, #12015, #27468, #22484, #6867, #17346, #27809, #4293, #24392, #866, #18040, #4466, #4806, #25579, #15285, #23353, #2227, #2409, #33289, #33110, #7382, #27979, #4636, #12704, #17518, #9961 ),
 .UNSPECIFIED., .F., .T. ) 
 B_SPLINE_CURVE_WITH_KNOTS ( ( 3, 2, 2, 2, 2, 2, 2, 2, 2, 2, 2, 2, 2, 2, 2, 2, 2, 2, 2, 2, 2, 2, 2, 2, 2, 2, 2, 2, 2, 2, 2, 2, 2, 2, 2, 2, 2, 3 ),
 ( 0.000000000000000000, 0.02000000000000000042, 0.04000000000000000083, 0.05999999999999999778, 0.08000000000000000167, 0.1000000000000000056, 0.1199999999999999956, 0.1400000000000000133, 0.1600000000000000033, 0.1799999999999999933, 0.2000000000000000111, 0.2200000000000000011, 0.2399999999999999911, 0.2600000000000000089, 0.2800000000000000266, 0.2999999999999999889, 0.3200000000000000067, 0.3400000000000000244, 0.3599999999999999867, 0.3800000000000000044, 0.4000000000000000222, 0.4199999999999999845, 0.4400000000000000022, 0.4600000000000000200, 0.4799999999999999822, 0.5000000000000000000, 0.5200000000000000178, 0.5400000000000000355, 0.5600000000000000533, 0.5799999999999999600, 0.5999999999999999778, 0.6199999999999999956, 0.6400000000000000133, 0.6600000000000000311, 0.6800000000000000488, 0.6999999999999999556, 0.7199999999999999734, 0.7374174419963591687 ),
 .UNSPECIFIED. ) 
 CURVE ( )  GEOMETRIC_REPRESENTATION_ITEM ( )  RATIONAL_B_SPLINE_CURVE ( ( 1.000000000000000000, 0.9510565162951535312, 1.000000000000000000, 0.9510565162951535312, 1.000000000000000000, 0.9510565162951535312, 1.000000000000000000, 0.9510565162951535312, 1.000000000000000000, 0.9510565162951535312, 1.000000000000000000, 0.9510565162951535312, 1.000000000000000000, 0.9510565162951535312, 1.000000000000000000, 0.9510565162951535312, 1.000000000000000000, 0.9510565162951535312, 1.000000000000000000, 0.9510565162951535312, 1.000000000000000000, 0.9510565162951535312, 1.000000000000000000, 0.9510565162951535312, 1.000000000000000000, 0.9510565162951535312, 1.000000000000000000, 0.9510565162951535312, 1.000000000000000000, 0.9510565162951535312, 1.000000000000000000, 0.9510565162951535312, 1.000000000000000000, 0.9510565162951535312, 1.000000000000000000, 0.9510565162951535312, 1.000000000000000000, 0.9510565162951535312, 1.000000000000000000, 0.9510565162951535312, 1.000000000000000000, 0.9510565162951535312, 1.000000000000000000, 0.9510565162951535312, 1.000000000000000000, 0.9510565162951535312, 1.000000000000000000, 0.9510565162951535312, 1.000000000000000000, 0.9510565162951535312, 1.000000000000000000, 0.9510565162951535312, 1.000000000000000000, 0.9510565162951535312, 1.000000000000000000, 0.9510565162951535312, 1.000000000000000000, 0.9510565162951535312, 1.000000000000000000, 0.9510565162951535312, 1.000000000000000000, 0.9510565162951535312, 1.000000000000000000, 0.9510565162951535312, 1.000000000000000000, 0.9510565162951535312, 1.000000000000000000, 0.9510565162951535312, 1.000000000000000000, 0.9510565162951535312, 1.000000000000000000, 0.9510565162951535312, 1.000000000000000000, 0.9573764855735540369, 0.9889922301674687333 ) ) 
 REPRESENTATION_ITEM ( '' )  );
#33013=DIRECTION ( 'NONE',  ( 0.000000000000000000, 1.000000000000000000, 0.000000000000000000 ) ) ;
#33024=CARTESIAN_POINT ( 'NONE',  ( 11.25946833292375793, 72.07500000273120122, -8.180482586598735395 ) ) ;
#33028=AXIS2_PLACEMENT_3D ( 'NONE', #14506, #9691, #7283 ) ;
#33057=CARTESIAN_POINT ( 'NONE',  ( -3.054597574617877509, 74.00000000000002842, 13.92607879720974218 ) ) ;
#33063=CARTESIAN_POINT ( 'NONE',  ( -1.467220197368425466E-15, 122.0000000000000000, -10.64101615137753676 ) ) ;
#33079=AXIS2_PLACEMENT_3D ( 'NONE', #15177, #22894, #32992 ) ;
#33100=CARTESIAN_POINT ( 'NONE',  ( 11.25946833292375793, 72.17500000273119554, 8.180482586598731842 ) ) ;
#33110=CARTESIAN_POINT ( 'NONE',  ( 11.25946833292375793, 74.57500000273120122, -8.180482586598735395 ) ) ;
#33112=CARTESIAN_POINT ( 'NONE',  ( 15.00000000000000355, 79.15000000546235981, 4.873795443493592394 ) ) ;
#33117=CARTESIAN_POINT ( 'NONE',  ( -12.13525491562421088, 74.05000000546240813, -8.816778784387096835 ) ) ;
#33124=CARTESIAN_POINT ( 'NONE',  ( 4.300734207923761154, 75.47500000273116427, 13.23629886949340495 ) ) ;
#33159=DIRECTION ( 'NONE',  ( -1.000000000000000000, 0.000000000000000000, 0.000000000000000000 ) ) ;
#33182=ORIENTED_EDGE ( 'NONE', *, *, #29912, .F. ) ;
#33183=AXIS2_PLACEMENT_3D ( 'NONE', #17179, #19246, #29522 ) ;
#33184=PLANE ( 'NONE',  #3437 ) ;
#33218=ORIENTED_EDGE ( 'NONE', *, *, #20072, .F. ) ;
#33232=CARTESIAN_POINT ( 'NONE',  ( -12.49601229055796914, 74.00000000000005684, 7.815062094324783715 ) ) ;
#33247=EDGE_CURVE ( 'NONE', #20845, #17411, #8547, .T. ) ;
#33258=CARTESIAN_POINT ( 'NONE',  ( -11.54700538379251995, 86.00000000000001421, -19.99999999999999645 ) ) ;
#33271=ORIENTED_EDGE ( 'NONE', *, *, #24474, .T. ) ;
#33279=CARTESIAN_POINT ( 'NONE',  ( 12.13525491562421088, 78.80000000000003979, 8.816778784387095058 ) ) ;
#33289=CARTESIAN_POINT ( 'NONE',  ( 8.601468415847516980, 74.67500000273120975, -11.83890561707634603 ) ) ;
#33291=CARTESIAN_POINT ( 'NONE',  ( -9.270509831248425314, 77.95000000546239960, -12.75976212528059861 ) ) ;
#33305=CARTESIAN_POINT ( 'NONE',  ( 8.601468415847516980, 80.67500000273118133, -11.83890561707634781 ) ) ;
#33309=CARTESIAN_POINT ( 'NONE',  ( 15.00000000000000000, 79.00000000000001421, -1.836970198721029589E-15 ) ) ;
#33312=ORIENTED_EDGE ( 'NONE', *, *, #11586, .F. ) ;
#33337=DIRECTION ( 'NONE',  ( 0.8660254037844388186, -0.000000000000000000, 0.4999999999999997780 ) ) ;
#33351=FACE_BOUND ( 'NONE', #10367, .T. ) ;
#33359=ORIENTED_EDGE ( 'NONE', *, *, #29363, .T. ) ;
#33361=CARTESIAN_POINT ( 'NONE',  ( -4.223320258572821363E-15, 80.50000000000001421, 15.00000000000000355 ) ) ;
#33379=CARTESIAN_POINT ( 'NONE',  ( 2.375766604868046361, 74.55125428154681799, 14.99999999999999822 ) ) ;
#33409=CARTESIAN_POINT ( 'NONE',  ( 0.000000000000000000, 111.9999999999999858, 11.32050807568876749 ) ) ;
#33410=CARTESIAN_POINT ( 'NONE',  ( 4.250625530119172879, 74.00000000000000000, 13.31398618829670788 ) ) ;
#33418=CARTESIAN_POINT ( 'NONE',  ( -11.54700538379251817, 86.00000000000001421, 19.99999999999999645 ) ) ;
#33443=ORIENTED_EDGE ( 'NONE', *, *, #31596, .F. ) ;
#33447=CARTESIAN_POINT ( 'NONE',  ( 11.54700538379251817, 96.00000000000002842, 19.99999999999999645 ) ) ;
#33449=CARTESIAN_POINT ( 'NONE',  ( 4.635254915624212657, 78.85000000546239107, 14.26584774442730286 ) ) ;
#33452=CARTESIAN_POINT ( 'NONE',  ( -9.270509831248421762, 76.30000000000003979, 12.75976212528060039 ) ) ;
#33463=CARTESIAN_POINT ( 'NONE',  ( -15.00000000000000000, 74.35000000546239107, 4.873795443493597723 ) ) ;
#33464=CARTESIAN_POINT ( 'NONE',  ( 23.09401076758502569, 86.00000000000001421, -6.857326241137392698E-15 ) ) ;
#33476=CARTESIAN_POINT ( 'NONE',  ( -8.601468415847518756, 81.07500000273115859, -11.83890561707634781 ) ) ;
#33529=CYLINDRICAL_SURFACE ( 'NONE', #2578, 15.00000000000000000 ) ;
#33532=EDGE_LOOP ( 'NONE', ( #33705, #22263, #11551, #20288 ) ) ;
#33540=LINE ( 'NONE', #23079, #2929 ) ;
#33545=CARTESIAN_POINT ( 'NONE',  ( 0.000000000000000000, 111.9999999999999858, 0.000000000000000000 ) ) ;
#33547=DIRECTION ( 'NONE',  ( 0.000000000000000000, -0.000000000000000000, 1.000000000000000000 ) ) ;
#33557=ADVANCED_FACE ( 'NONE', ( #14882 ), #25521, .T. ) ;
#33574=CARTESIAN_POINT ( 'NONE',  ( 0.000000000000000000, 111.9999999999999858, 0.000000000000000000 ) ) ;
#33576=DIRECTION ( 'NONE',  ( 0.000000000000000000, 0.000000000000000000, -1.000000000000000000 ) ) ;
#33623=CARTESIAN_POINT ( 'NONE',  ( 15.00000000000000000, 79.25000000546239676, -1.836970198721029589E-15 ) ) ;
#33626=CARTESIAN_POINT ( 'NONE',  ( 2.897257156509938333E-15, 76.50000000000002842, 15.77193336357400710 ) ) ;
#33639=CARTESIAN_POINT ( 'NONE',  ( 12.13525491562421088, 73.05000000546240813, 8.816778784387095058 ) ) ;
#33649=CARTESIAN_POINT ( 'NONE',  ( -9.270509831248423538, 81.69999999999997442, -12.75976212528059861 ) ) ;
#33652=CARTESIAN_POINT ( 'NONE',  ( -13.91746824999999532, 75.47500000273116427, 4.522059556121122093 ) ) ;
#33705=ORIENTED_EDGE ( 'NONE', *, *, #6564, .F. ) ;
#33715=ORIENTED_EDGE ( 'NONE', *, *, #2822, .F. ) ;
#33733=CARTESIAN_POINT ( 'NONE',  ( 13.91746824999999887, 71.87500000273122680, -1.704398294459741270E-15 ) ) ;
#33750=CIRCLE ( 'NONE', #26443, 13.32050807568876927 ) ;
#33805=CARTESIAN_POINT ( 'NONE',  ( 4.635254915624212657, 78.60000000000000853, 14.26584774442730286 ) ) ;
#33823=CARTESIAN_POINT ( 'NONE',  ( -4.300734207923755825, 75.27500000273118985, 13.23629886949340673 ) ) ;
#33826=CARTESIAN_POINT ( 'NONE',  ( -13.91746824999999887, 77.37500000273116996, 0.000000000000000000 ) ) ;
#33876=CARTESIAN_POINT ( 'NONE',  ( -11.54700538379251995, 96.00000000000002842, -19.99999999999999645 ) ) ;
#33895=ADVANCED_FACE ( 'NONE', ( #26629 ), #27697, .T. ) ;
#33907=ADVANCED_FACE ( 'NONE', ( #18748 ), #5355, .F. ) ;
#33913=EDGE_CURVE ( 'NONE', #16375, #26497, #10765, .T. ) ;
#33968=CARTESIAN_POINT ( 'NONE',  ( -15.00000000000000000, 74.09999999999999432, 4.873795443493597723 ) ) ;
#33971=LINE ( 'NONE', #31392, #19791 ) ;
#33979=CARTESIAN_POINT ( 'NONE',  ( -6.668671393434016714, 74.00000000000001421, -13.28991759065290168 ) ) ;
ENDSEC;
END-ISO-10303-21;
